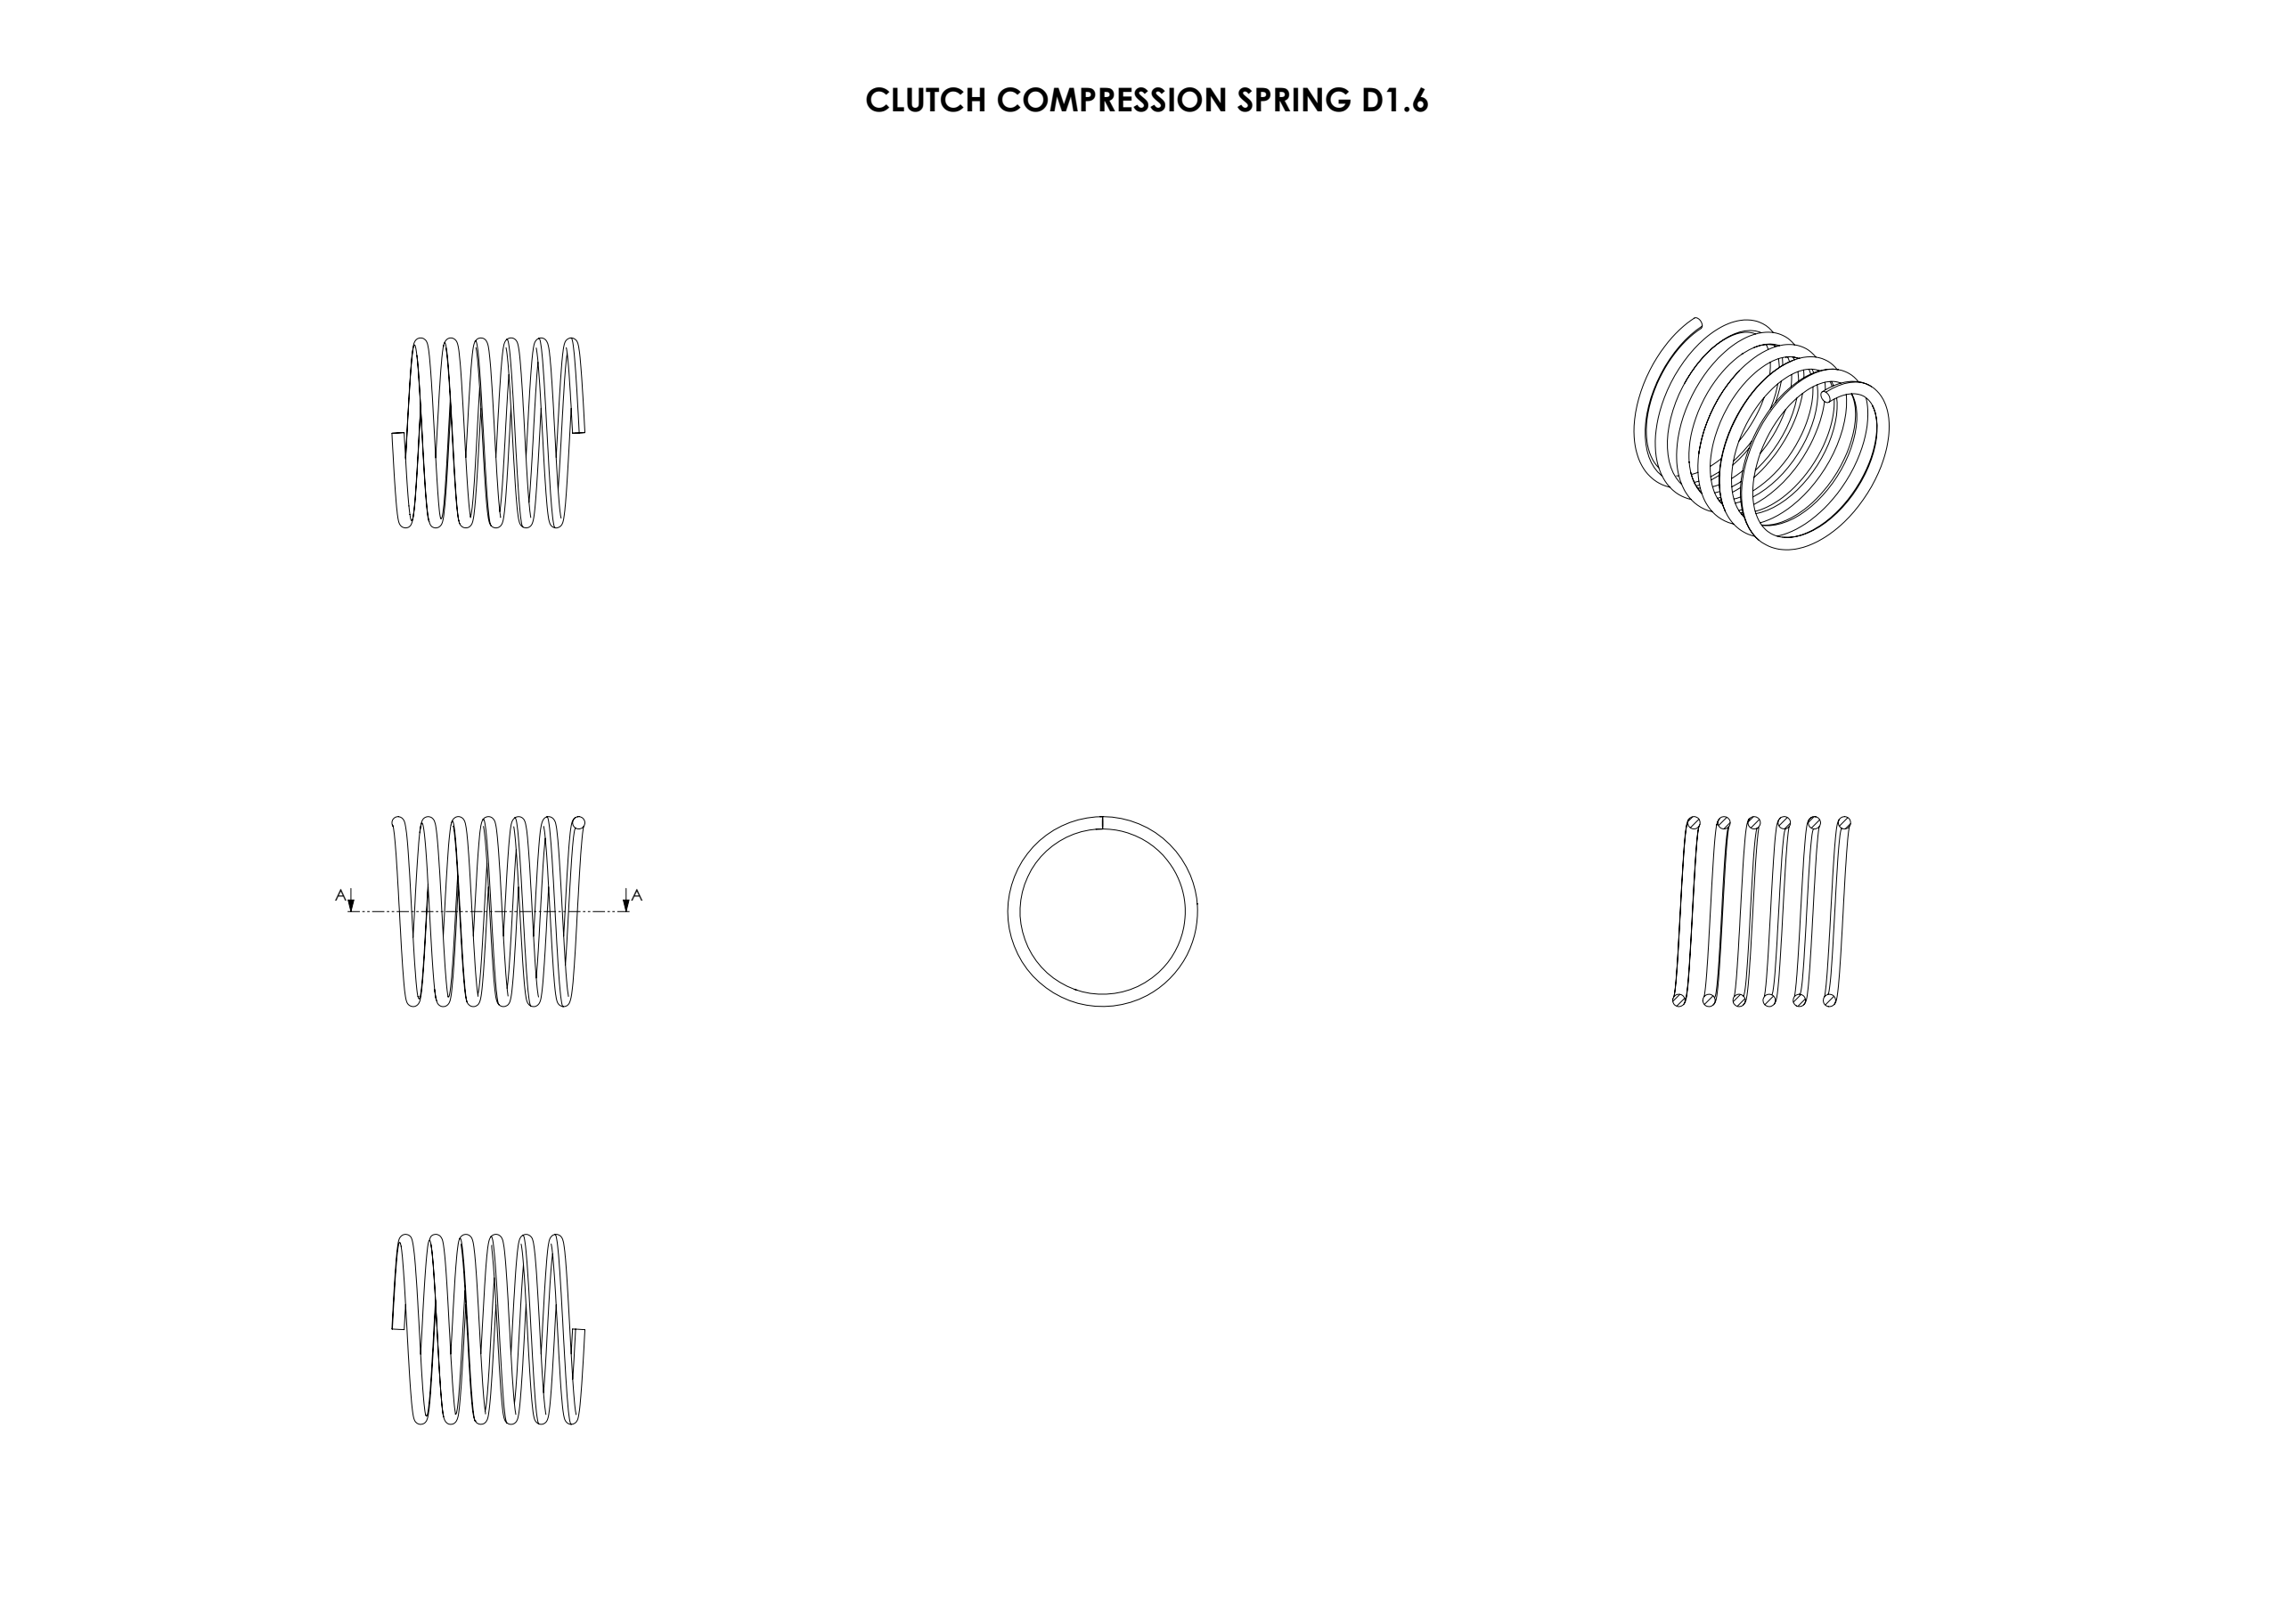
ISO-10303-21;
HEADER;
/* Generated by software containing ST-Developer
 * from STEP Tools, Inc. (www.steptools.com) 
 */

FILE_DESCRIPTION(
/* description */ (''),
/* implementation_level */ '2;1');

FILE_NAME(
/* name */ '10_Clutch_Compression_Spring_d1.6.step',
/* time_stamp */ '2026-10-11T13:00:10-07:00',
/* author */ (''),
/* organization */ (''),
/* preprocessor_version */ 'ST-DEVELOPER v20.2',
/* originating_system */ 'Autodesk Translation Framework v15.15.0.0',
/* authorisation */ '');

FILE_SCHEMA (('AUTOMOTIVE_DESIGN { 1 0 10303 214 3 1 1 }'));
ENDSEC;

DATA;
#10=MECHANICAL_DESIGN_GEOMETRIC_PRESENTATION_REPRESENTATION('',(#367),#65563);
#345=SHAPE_REPRESENTATION_RELATIONSHIP('SRR','None',#65623,#356);
#356=ADVANCED_BREP_SHAPE_REPRESENTATION('',(#378),#65561);
#367=STYLED_ITEM('',(#65788),#378);
#378=MANIFOLD_SOLID_BREP('Body1',#20017);
#843=B_SPLINE_SURFACE_WITH_KNOTS('',3,3,((#62685,#62686,#62687,#62688,#62689,
#62690,#62691,#62692,#62693,#62694,#62695,#62696,#62697,#62698,#62699,#62700,
#62701,#62702,#62703,#62704,#62705,#62706,#62707,#62708,#62709,#62710,#62711,
#62712,#62713,#62714,#62715,#62716,#62717,#62718,#62719,#62720,#62721,#62722,
#62723,#62724,#62725,#62726,#62727,#62728,#62729,#62730,#62731,#62732,#62733,
#62734,#62735,#62736,#62737,#62738,#62739,#62740,#62741,#62742,#62743,#62744,
#62745,#62746,#62747,#62748,#62749,#62750,#62751,#62752,#62753,#62754,#62755,
#62756,#62757,#62758,#62759,#62760),(#62761,#62762,#62763,#62764,#62765,
#62766,#62767,#62768,#62769,#62770,#62771,#62772,#62773,#62774,#62775,#62776,
#62777,#62778,#62779,#62780,#62781,#62782,#62783,#62784,#62785,#62786,#62787,
#62788,#62789,#62790,#62791,#62792,#62793,#62794,#62795,#62796,#62797,#62798,
#62799,#62800,#62801,#62802,#62803,#62804,#62805,#62806,#62807,#62808,#62809,
#62810,#62811,#62812,#62813,#62814,#62815,#62816,#62817,#62818,#62819,#62820,
#62821,#62822,#62823,#62824,#62825,#62826,#62827,#62828,#62829,#62830,#62831,
#62832,#62833,#62834,#62835,#62836),(#62837,#62838,#62839,#62840,#62841,
#62842,#62843,#62844,#62845,#62846,#62847,#62848,#62849,#62850,#62851,#62852,
#62853,#62854,#62855,#62856,#62857,#62858,#62859,#62860,#62861,#62862,#62863,
#62864,#62865,#62866,#62867,#62868,#62869,#62870,#62871,#62872,#62873,#62874,
#62875,#62876,#62877,#62878,#62879,#62880,#62881,#62882,#62883,#62884,#62885,
#62886,#62887,#62888,#62889,#62890,#62891,#62892,#62893,#62894,#62895,#62896,
#62897,#62898,#62899,#62900,#62901,#62902,#62903,#62904,#62905,#62906,#62907,
#62908,#62909,#62910,#62911,#62912),(#62913,#62914,#62915,#62916,#62917,
#62918,#62919,#62920,#62921,#62922,#62923,#62924,#62925,#62926,#62927,#62928,
#62929,#62930,#62931,#62932,#62933,#62934,#62935,#62936,#62937,#62938,#62939,
#62940,#62941,#62942,#62943,#62944,#62945,#62946,#62947,#62948,#62949,#62950,
#62951,#62952,#62953,#62954,#62955,#62956,#62957,#62958,#62959,#62960,#62961,
#62962,#62963,#62964,#62965,#62966,#62967,#62968,#62969,#62970,#62971,#62972,
#62973,#62974,#62975,#62976,#62977,#62978,#62979,#62980,#62981,#62982,#62983,
#62984,#62985,#62986,#62987,#62988),(#62989,#62990,#62991,#62992,#62993,
#62994,#62995,#62996,#62997,#62998,#62999,#63000,#63001,#63002,#63003,#63004,
#63005,#63006,#63007,#63008,#63009,#63010,#63011,#63012,#63013,#63014,#63015,
#63016,#63017,#63018,#63019,#63020,#63021,#63022,#63023,#63024,#63025,#63026,
#63027,#63028,#63029,#63030,#63031,#63032,#63033,#63034,#63035,#63036,#63037,
#63038,#63039,#63040,#63041,#63042,#63043,#63044,#63045,#63046,#63047,#63048,
#63049,#63050,#63051,#63052,#63053,#63054,#63055,#63056,#63057,#63058,#63059,
#63060,#63061,#63062,#63063,#63064),(#63065,#63066,#63067,#63068,#63069,
#63070,#63071,#63072,#63073,#63074,#63075,#63076,#63077,#63078,#63079,#63080,
#63081,#63082,#63083,#63084,#63085,#63086,#63087,#63088,#63089,#63090,#63091,
#63092,#63093,#63094,#63095,#63096,#63097,#63098,#63099,#63100,#63101,#63102,
#63103,#63104,#63105,#63106,#63107,#63108,#63109,#63110,#63111,#63112,#63113,
#63114,#63115,#63116,#63117,#63118,#63119,#63120,#63121,#63122,#63123,#63124,
#63125,#63126,#63127,#63128,#63129,#63130,#63131,#63132,#63133,#63134,#63135,
#63136,#63137,#63138,#63139,#63140),(#63141,#63142,#63143,#63144,#63145,
#63146,#63147,#63148,#63149,#63150,#63151,#63152,#63153,#63154,#63155,#63156,
#63157,#63158,#63159,#63160,#63161,#63162,#63163,#63164,#63165,#63166,#63167,
#63168,#63169,#63170,#63171,#63172,#63173,#63174,#63175,#63176,#63177,#63178,
#63179,#63180,#63181,#63182,#63183,#63184,#63185,#63186,#63187,#63188,#63189,
#63190,#63191,#63192,#63193,#63194,#63195,#63196,#63197,#63198,#63199,#63200,
#63201,#63202,#63203,#63204,#63205,#63206,#63207,#63208,#63209,#63210,#63211,
#63212,#63213,#63214,#63215,#63216),(#63217,#63218,#63219,#63220,#63221,
#63222,#63223,#63224,#63225,#63226,#63227,#63228,#63229,#63230,#63231,#63232,
#63233,#63234,#63235,#63236,#63237,#63238,#63239,#63240,#63241,#63242,#63243,
#63244,#63245,#63246,#63247,#63248,#63249,#63250,#63251,#63252,#63253,#63254,
#63255,#63256,#63257,#63258,#63259,#63260,#63261,#63262,#63263,#63264,#63265,
#63266,#63267,#63268,#63269,#63270,#63271,#63272,#63273,#63274,#63275,#63276,
#63277,#63278,#63279,#63280,#63281,#63282,#63283,#63284,#63285,#63286,#63287,
#63288,#63289,#63290,#63291,#63292),(#63293,#63294,#63295,#63296,#63297,
#63298,#63299,#63300,#63301,#63302,#63303,#63304,#63305,#63306,#63307,#63308,
#63309,#63310,#63311,#63312,#63313,#63314,#63315,#63316,#63317,#63318,#63319,
#63320,#63321,#63322,#63323,#63324,#63325,#63326,#63327,#63328,#63329,#63330,
#63331,#63332,#63333,#63334,#63335,#63336,#63337,#63338,#63339,#63340,#63341,
#63342,#63343,#63344,#63345,#63346,#63347,#63348,#63349,#63350,#63351,#63352,
#63353,#63354,#63355,#63356,#63357,#63358,#63359,#63360,#63361,#63362,#63363,
#63364,#63365,#63366,#63367,#63368),(#63369,#63370,#63371,#63372,#63373,
#63374,#63375,#63376,#63377,#63378,#63379,#63380,#63381,#63382,#63383,#63384,
#63385,#63386,#63387,#63388,#63389,#63390,#63391,#63392,#63393,#63394,#63395,
#63396,#63397,#63398,#63399,#63400,#63401,#63402,#63403,#63404,#63405,#63406,
#63407,#63408,#63409,#63410,#63411,#63412,#63413,#63414,#63415,#63416,#63417,
#63418,#63419,#63420,#63421,#63422,#63423,#63424,#63425,#63426,#63427,#63428,
#63429,#63430,#63431,#63432,#63433,#63434,#63435,#63436,#63437,#63438,#63439,
#63440,#63441,#63442,#63443,#63444)),.UNSPECIFIED.,.T.,.F.,.F.,(4,1,1,1,
1,1,1,4),(4,1,1,1,1,1,1,1,1,1,1,1,1,1,1,1,1,1,1,1,1,1,1,1,1,1,1,1,1,1,1,
1,1,1,1,1,1,1,1,1,1,1,1,1,1,1,1,1,1,1,1,1,1,1,1,1,1,1,1,1,1,1,1,1,1,1,1,
1,1,1,1,1,1,4),(-3.14159265358979,-2.24399475256414,-1.34639685153848,-0.448798950512828,
0.448798950512828,1.34639685153848,2.24399475256414,3.14159265358979),(0.,
0.00892857142857143,0.0178571428571429,0.0357142857142857,0.0535714285714286,
0.0714285714285714,0.0892857142857143,0.107142857142857,0.125,0.142857142857143,
0.158730158730159,0.174603174603175,0.182539682539683,0.186507936507937,
0.19047619047619,0.202380952380952,0.214285714285714,0.226190476190476,
0.238095238095238,0.25,0.261904761904762,0.273809523809524,0.279761904761905,
0.285714285714286,0.297619047619048,0.30952380952381,0.321428571428571,
0.333333333333333,0.349206349206349,0.365079365079365,0.380952380952381,
0.396825396825397,0.412698412698413,0.428571428571429,0.436507936507937,
0.452380952380952,0.464285714285714,0.476190476190476,0.488095238095238,
0.5,0.517857142857143,0.535714285714286,0.553571428571429,0.571428571428571,
0.589285714285714,0.607142857142857,0.625,0.642857142857143,0.651785714285714,
0.660714285714286,0.678571428571428,0.696428571428571,0.714285714285714,
0.726190476190476,0.738095238095238,0.75,0.761904761904762,0.773809523809524,
0.785714285714286,0.797619047619047,0.809523809523809,0.821428571428571,
0.833333333333333,0.845238095238095,0.857142857142857,0.875,0.892857142857143,
0.910714285714286,0.928571428571429,0.946428571428571,0.964285714285714,
0.982142857142857,0.991071428571429,1.),.UNSPECIFIED.);
#1038=PLANE('',#22039);
#1039=PLANE('',#22040);
#2148=FACE_OUTER_BOUND('',#3376,.T.);
#2149=FACE_OUTER_BOUND('',#3377,.T.);
#2150=FACE_OUTER_BOUND('',#3378,.T.);
#3376=EDGE_LOOP('',(#17434,#17435,#17436,#17437));
#3377=EDGE_LOOP('',(#17438));
#3378=EDGE_LOOP('',(#17439));
#4481=CIRCLE('',#22037,0.8);
#4482=CIRCLE('',#22038,0.8);
#5356=B_SPLINE_CURVE_WITH_KNOTS('',3,(#63448,#63449,#63450,#63451,#63452,
#63453,#63454,#63455,#63456,#63457,#63458,#63459,#63460,#63461,#63462,#63463,
#63464,#63465,#63466,#63467,#63468,#63469,#63470,#63471,#63472,#63473,#63474,
#63475,#63476,#63477,#63478,#63479,#63480,#63481,#63482,#63483,#63484,#63485,
#63486,#63487,#63488,#63489,#63490,#63491,#63492,#63493,#63494,#63495,#63496,
#63497,#63498,#63499,#63500,#63501,#63502,#63503,#63504,#63505,#63506,#63507,
#63508,#63509,#63510,#63511,#63512,#63513,#63514,#63515,#63516,#63517,#63518,
#63519,#63520,#63521,#63522,#63523),.UNSPECIFIED.,.F.,.F.,(4,1,1,1,1,1,
1,1,1,1,1,1,1,1,1,1,1,1,1,1,1,1,1,1,1,1,1,1,1,1,1,1,1,1,1,1,1,1,1,1,1,1,
1,1,1,1,1,1,1,1,1,1,1,1,1,1,1,1,1,1,1,1,1,1,1,1,1,1,1,1,1,1,1,4),(0.,0.00892857142857143,
0.0178571428571429,0.0357142857142857,0.0535714285714286,0.0714285714285714,
0.0892857142857143,0.107142857142857,0.125,0.142857142857143,0.158730158730159,
0.174603174603175,0.182539682539683,0.186507936507937,0.19047619047619,
0.202380952380952,0.214285714285714,0.226190476190476,0.238095238095238,
0.25,0.261904761904762,0.273809523809524,0.279761904761905,0.285714285714286,
0.297619047619048,0.30952380952381,0.321428571428571,0.333333333333333,
0.349206349206349,0.365079365079365,0.380952380952381,0.396825396825397,
0.412698412698413,0.428571428571429,0.436507936507937,0.452380952380952,
0.464285714285714,0.476190476190476,0.488095238095238,0.5,0.517857142857143,
0.535714285714286,0.553571428571429,0.571428571428571,0.589285714285714,
0.607142857142857,0.625,0.642857142857143,0.651785714285714,0.660714285714286,
0.678571428571428,0.696428571428571,0.714285714285714,0.726190476190476,
0.738095238095238,0.75,0.761904761904762,0.773809523809524,0.785714285714286,
0.797619047619047,0.809523809523809,0.821428571428571,0.833333333333333,
0.845238095238095,0.857142857142857,0.875,0.892857142857143,0.910714285714286,
0.928571428571429,0.946428571428571,0.964285714285714,0.982142857142857,
0.991071428571429,1.),.UNSPECIFIED.);
#8857=VERTEX_POINT('',#63445);
#8858=VERTEX_POINT('',#63447);
#11750=EDGE_CURVE('',#8857,#8857,#4481,.T.);
#11751=EDGE_CURVE('',#8857,#8858,#5356,.T.);
#11752=EDGE_CURVE('',#8858,#8858,#4482,.T.);
#17434=ORIENTED_EDGE('',*,*,#11750,.T.);
#17435=ORIENTED_EDGE('',*,*,#11751,.T.);
#17436=ORIENTED_EDGE('',*,*,#11752,.F.);
#17437=ORIENTED_EDGE('',*,*,#11751,.F.);
#17438=ORIENTED_EDGE('',*,*,#11752,.T.);
#17439=ORIENTED_EDGE('',*,*,#11750,.F.);
#19844=ADVANCED_FACE('',(#2148),#843,.T.);
#19845=ADVANCED_FACE('',(#2149),#1038,.T.);
#19846=ADVANCED_FACE('',(#2150),#1039,.F.);
#20017=CLOSED_SHELL('',(#19844,#19845,#19846));
#22036=AXIS2_PLACEMENT_3D('',#62684,#26929,#26930);
#22037=AXIS2_PLACEMENT_3D('',#63446,#26931,#26932);
#22038=AXIS2_PLACEMENT_3D('',#63524,#26933,#26934);
#22039=AXIS2_PLACEMENT_3D('',#63525,#26935,#26936);
#22040=AXIS2_PLACEMENT_3D('',#63526,#26937,#26938);
#26929=DIRECTION('axis',(0.,0.,1.));
#26930=DIRECTION('refdir',(1.,0.,0.));
#26931=DIRECTION('center_axis',(0.0524864875083004,-0.00359342805144231,
0.998615169073593));
#26932=DIRECTION('ref_axis',(-0.996282959525764,0.0682093869087291,0.052609353694185));
#26933=DIRECTION('center_axis',(0.052486487479681,0.00359342804742538,0.998615169075111));
#26934=DIRECTION('ref_axis',(0.504066799442469,0.863157308043356,-0.029599379574115));
#26935=DIRECTION('center_axis',(0.052486487479681,0.00359342804742538,0.998615169075111));
#26936=DIRECTION('ref_axis',(0.504066799442469,0.863157308043356,-0.029599379574115));
#26937=DIRECTION('center_axis',(0.0524864875083004,-0.00359342805144231,
0.998615169073593));
#26938=DIRECTION('ref_axis',(-0.996282959525764,0.0682093869087291,0.052609353694185));
#62684=CARTESIAN_POINT('',(0.,0.,0.));
#62685=CARTESIAN_POINT('Ctrl Pts',(-5.40297363237939,11.445432490473,-0.042087482955348));
#62686=CARTESIAN_POINT('Ctrl Pts',(-5.33369696111111,11.4406895414653,1.27598004405306));
#62687=CARTESIAN_POINT('Ctrl Pts',(-5.19521862607164,11.0085774465653,3.79612986924071));
#62688=CARTESIAN_POINT('Ctrl Pts',(-4.91840015088629,8.49992872694836,8.36573269447326));
#62689=CARTESIAN_POINT('Ctrl Pts',(-4.57320339639667,2.77438806679843,11.967805106163));
#62690=CARTESIAN_POINT('Ctrl Pts',(-4.15990469688328,-5.28321395100969,
11.056569093912));
#62691=CARTESIAN_POINT('Ctrl Pts',(-3.747686811287,-10.9955419925911,5.33820880446098));
#62692=CARTESIAN_POINT('Ctrl Pts',(-3.33647538038886,-11.8953437286105,
-2.67607624391012));
#62693=CARTESIAN_POINT('Ctrl Pts',(-2.92629230091383,-7.61357058494829,
-9.48509907357355));
#62694=CARTESIAN_POINT('Ctrl Pts',(-2.51711411539744,-0.0352081461009456,
-12.133141923791));
#62695=CARTESIAN_POINT('Ctrl Pts',(-2.12405346851776,7.23325257089384,-9.58201967934875));
#62696=CARTESIAN_POINT('Ctrl Pts',(-1.74697035839629,11.3507348234515,-3.53593739186965));
#62697=CARTESIAN_POINT('Ctrl Pts',(-1.44594495704173,11.3410956049915,2.29151330201399));
#62698=CARTESIAN_POINT('Ctrl Pts',(-1.23555813837642,9.62414272926665,5.84190263222694));
#62699=CARTESIAN_POINT('Ctrl Pts',(-1.11543119956109,8.23345778533256,7.58643680207061));
#62700=CARTESIAN_POINT('Ctrl Pts',(-0.965350761047819,6.18988758696103,
9.48427609552777));
#62701=CARTESIAN_POINT('Ctrl Pts',(-0.755455752947343,2.59800826091561,
11.2146857757666));
#62702=CARTESIAN_POINT('Ctrl Pts',(-0.486005297879084,-2.52226170629262,
11.2131697972667));
#62703=CARTESIAN_POINT('Ctrl Pts',(-0.216964169512981,-7.12771226807027,
8.99614845847778));
#62704=CARTESIAN_POINT('Ctrl Pts',(0.051673199605982,-10.3093017586739,
5.0037967419436));
#62705=CARTESIAN_POINT('Ctrl Pts',(0.319912004204202,-11.4424452984132,
0.0352862821531482));
#62706=CARTESIAN_POINT('Ctrl Pts',(0.587759827560524,-10.3093945561263,
-4.92692882386994));
#62707=CARTESIAN_POINT('Ctrl Pts',(0.810644510337,-7.66768866486485,-8.23632315062337));
#62708=CARTESIAN_POINT('Ctrl Pts',(0.9887628738834,-4.85431418623128,-10.0009017448057));
#62709=CARTESIAN_POINT('Ctrl Pts',(1.16675569936477,-1.72248496421437,-11.0992889627176));
#62710=CARTESIAN_POINT('Ctrl Pts',(1.38901397173341,2.49959534000996,-11.0999021750131));
#62711=CARTESIAN_POINT('Ctrl Pts',(1.65535913685916,7.06073570919373,-8.90264472811187));
#62712=CARTESIAN_POINT('Ctrl Pts',(1.92134523430893,10.2082911979719,-4.95142581114747));
#62713=CARTESIAN_POINT('Ctrl Pts',(2.21649491340346,11.464268710378,0.517623581655109));
#62714=CARTESIAN_POINT('Ctrl Pts',(2.54067136572795,9.61231028484355,6.51924754582076));
#62715=CARTESIAN_POINT('Ctrl Pts',(2.89372530199723,4.26040343756882,10.7809878391944));
#62716=CARTESIAN_POINT('Ctrl Pts',(3.24620579430313,-2.5499807271206,11.2895594263092));
#62717=CARTESIAN_POINT('Ctrl Pts',(3.59813519099429,-8.45086172951072,7.88046583695986));
#62718=CARTESIAN_POINT('Ctrl Pts',(3.94952923360969,-11.4105207073045,1.7432987177926));
#62719=CARTESIAN_POINT('Ctrl Pts',(4.24193167813174,-10.5600221745821,-3.85384587814088));
#62720=CARTESIAN_POINT('Ctrl Pts',(4.53402805814432,-7.47314001623606,-8.38031426693708));
#62721=CARTESIAN_POINT('Ctrl Pts',(4.79664370266186,-3.07363708606063,-10.9230350253262));
#62722=CARTESIAN_POINT('Ctrl Pts',(5.08810557752102,2.47013445948664,-10.9134823314909));
#62723=CARTESIAN_POINT('Ctrl Pts',(5.35017440554513,6.95492422204958,-8.75633618182547));
#62724=CARTESIAN_POINT('Ctrl Pts',(5.61200361956877,10.0542035018942,-4.86537952153394));
#62725=CARTESIAN_POINT('Ctrl Pts',(5.91720482332597,11.3540414258911,0.789064544875747));
#62726=CARTESIAN_POINT('Ctrl Pts',(6.26564105547289,9.10553979339257,7.23636750926088));
#62727=CARTESIAN_POINT('Ctrl Pts',(6.65717646488775,2.59867870246558,11.321535036503));
#62728=CARTESIAN_POINT('Ctrl Pts',(7.04828730943666,-5.02094595929096,10.4607994583915));
#62729=CARTESIAN_POINT('Ctrl Pts',(7.43900933211819,-10.4395500322981,5.04208746732736));
#62730=CARTESIAN_POINT('Ctrl Pts',(7.82938055234697,-11.2946782793107,-2.56617594127693));
#62731=CARTESIAN_POINT('Ctrl Pts',(8.21943575999143,-7.22551638204153,-9.04156914965989));
#62732=CARTESIAN_POINT('Ctrl Pts',(8.60921106212656,-0.0075686889805855,
-11.5674090717167));
#62733=CARTESIAN_POINT('Ctrl Pts',(8.93382080129404,5.99528673196386,-9.45936192902959));
#62734=CARTESIAN_POINT('Ctrl Pts',(9.19340748731854,9.23614030177817,-5.81293639312917));
#62735=CARTESIAN_POINT('Ctrl Pts',(9.45293101808351,11.1142702697208,-1.3107448337562));
#62736=CARTESIAN_POINT('Ctrl Pts',(9.77723136794952,10.4154952826205,5.00401083523754));
#62737=CARTESIAN_POINT('Ctrl Pts',(10.1662605952158,5.00921490063267,10.4044353775234));
#62738=CARTESIAN_POINT('Ctrl Pts',(10.5119839322498,-1.72077939907436,11.154116840079));
#62739=CARTESIAN_POINT('Ctrl Pts',(10.8144567422258,-6.89887898300864,8.65022675987097));
#62740=CARTESIAN_POINT('Ctrl Pts',(11.0737061869649,-9.97097573622103,4.80256799145211));
#62741=CARTESIAN_POINT('Ctrl Pts',(11.332954454476,-11.0656005972151,-0.0012636146746602));
#62742=CARTESIAN_POINT('Ctrl Pts',(11.592212676988,-9.96981484505854,-4.80333442118138));
#62743=CARTESIAN_POINT('Ctrl Pts',(11.8514921790329,-6.89841951530921,-8.65513848120015));
#62744=CARTESIAN_POINT('Ctrl Pts',(12.1108041978391,-2.45923784927583,-10.7938299796143));
#62745=CARTESIAN_POINT('Ctrl Pts',(12.3701601255276,2.46836208123245,-10.7925664321256));
#62746=CARTESIAN_POINT('Ctrl Pts',(12.6295710107042,6.9094980637413,-8.65413386138286));
#62747=CARTESIAN_POINT('Ctrl Pts',(12.8890481983849,9.98316171476258,-4.8004177652554));
#62748=CARTESIAN_POINT('Ctrl Pts',(13.1486032818335,11.0817124894507,0.00909499825818533));
#62749=CARTESIAN_POINT('Ctrl Pts',(13.4082458776239,9.98216422539828,4.81540788001813));
#62750=CARTESIAN_POINT('Ctrl Pts',(13.7112804745406,6.39794424339377,9.32638055254148));
#62751=CARTESIAN_POINT('Ctrl Pts',(14.0577858522366,-0.00835395432331517,
11.5770141955486));
#62752=CARTESIAN_POINT('Ctrl Pts',(14.4478987172592,-7.23337005489467,9.04881838019601));
#62753=CARTESIAN_POINT('Ctrl Pts',(14.8383177312182,-11.3068424364633,2.56726391915326));
#62754=CARTESIAN_POINT('Ctrl Pts',(15.2291319944184,-10.4497082271469,-5.04888270590908));
#62755=CARTESIAN_POINT('Ctrl Pts',(15.6202557238013,-5.02806227013448,-10.4744930049956));
#62756=CARTESIAN_POINT('Ctrl Pts',(16.0119892870161,2.60831854215743,-11.3347514386656));
#62757=CARTESIAN_POINT('Ctrl Pts',(16.338482088023,8.02442066121112,-7.9277656209221));
#62758=CARTESIAN_POINT('Ctrl Pts',(16.6004710641513,10.3977390912262,-3.60280630418266));
#62759=CARTESIAN_POINT('Ctrl Pts',(16.7309850253063,10.8049718643827,-1.22750855798432));
#62760=CARTESIAN_POINT('Ctrl Pts',(16.796746560446,10.8094741535653,0.0236795036592751));
#62761=CARTESIAN_POINT('Ctrl Pts',(-5.38662443082758,11.6842329202395,-0.042087482955348));
#62762=CARTESIAN_POINT('Ctrl Pts',(-5.31602073284708,11.6793991178476,1.30122823777898));
#62763=CARTESIAN_POINT('Ctrl Pts',(-5.17453105309391,11.2378404310333,3.87611783187972));
#62764=CARTESIAN_POINT('Ctrl Pts',(-4.89207386432173,8.67783202920574,8.53871783783621));
#62765=CARTESIAN_POINT('Ctrl Pts',(-4.53961983973176,2.83264538933516,12.2168195484002));
#62766=CARTESIAN_POINT('Ctrl Pts',(-4.11779670190641,-5.39139693844397,
11.2859525558124));
#62767=CARTESIAN_POINT('Ctrl Pts',(-3.69704974086023,-11.2215827743621,
5.44988936613388));
#62768=CARTESIAN_POINT('Ctrl Pts',(-3.27740459014898,-12.1395545614036,
-2.72889999849327));
#62769=CARTESIAN_POINT('Ctrl Pts',(-2.8588531609028,-7.77040836600443,-9.67639362221006));
#62770=CARTESIAN_POINT('Ctrl Pts',(-2.44139968754143,-0.0388721142853535,
-12.3776586948657));
#62771=CARTESIAN_POINT('Ctrl Pts',(-2.04046215341628,7.3748814694369,-9.77518585108066));
#62772=CARTESIAN_POINT('Ctrl Pts',(-1.65589905289416,11.5736066792837,-3.60919969149015));
#62773=CARTESIAN_POINT('Ctrl Pts',(-1.34897071506894,11.563561957149,2.33231726086283));
#62774=CARTESIAN_POINT('Ctrl Pts',(-1.13450959748022,9.81333086311448,5.9513827672463));
#62775=CARTESIAN_POINT('Ctrl Pts',(-1.01206942024888,8.39587803284931,7.72948090408433));
#62776=CARTESIAN_POINT('Ctrl Pts',(-0.859108571001228,6.31309527913905,
9.66370587564346));
#62777=CARTESIAN_POINT('Ctrl Pts',(-0.645184736392552,2.65240388760526,
11.4271146010615));
#62778=CARTESIAN_POINT('Ctrl Pts',(-0.370635299740237,-2.5645957521349,
11.4254307821442));
#62779=CARTESIAN_POINT('Ctrl Pts',(-0.0965765947892482,-7.25574474773981,
9.16696825093226));
#62780=CARTESIAN_POINT('Ctrl Pts',(0.177029974179721,-10.495940553954,5.10090160620736));
#62781=CARTESIAN_POINT('Ctrl Pts',(0.450155222364603,-11.6494709439128,
0.0420395084777696));
#62782=CARTESIAN_POINT('Ctrl Pts',(0.722812894385383,-10.4960064731164,
-5.00904716447792));
#62783=CARTESIAN_POINT('Ctrl Pts',(0.949649833562332,-7.80748481493112,
-8.37685596577217));
#62784=CARTESIAN_POINT('Ctrl Pts',(1.13086935173756,-4.94518515744457,-10.1720883688267));
#62785=CARTESIAN_POINT('Ctrl Pts',(1.31193547259697,-1.75933863472017,-11.2893824118723));
#62786=CARTESIAN_POINT('Ctrl Pts',(1.53800808648294,2.53496041621199,-11.2898509308499));
#62787=CARTESIAN_POINT('Ctrl Pts',(1.80882928470653,7.17245519023224,-9.0555522803647));
#62788=CARTESIAN_POINT('Ctrl Pts',(2.07920370118388,10.3716655806418,-5.03925894158933));
#62789=CARTESIAN_POINT('Ctrl Pts',(2.37912972697024,11.6476623900761,0.518107830099377));
#62790=CARTESIAN_POINT('Ctrl Pts',(2.7084215266127,9.76615815837076,6.61394631540922));
#62791=CARTESIAN_POINT('Ctrl Pts',(3.06686380982559,4.33246375617594,10.9402548757315));
#62792=CARTESIAN_POINT('Ctrl Pts',(3.42458416068682,-2.57871836910459,11.4557472388598));
#62793=CARTESIAN_POINT('Ctrl Pts',(3.78156882350692,-8.56367510055875,7.99749077041819));
#62794=CARTESIAN_POINT('Ctrl Pts',(4.13779970244094,-11.5633896761636,1.77577652817538));
#62795=CARTESIAN_POINT('Ctrl Pts',(4.43407615107156,-10.7011768584388,-3.8951157658593));
#62796=CARTESIAN_POINT('Ctrl Pts',(4.72991998621853,-7.57473185360497,-8.4794174000976));
#62797=CARTESIAN_POINT('Ctrl Pts',(4.99579563816587,-3.12059647036658,-11.0531492863553));
#62798=CARTESIAN_POINT('Ctrl Pts',(5.29071945165254,2.48877066815634,-11.0432915057983));
#62799=CARTESIAN_POINT('Ctrl Pts',(5.55579786749363,7.02472382683712,-8.86124346251412));
#62800=CARTESIAN_POINT('Ctrl Pts',(5.82051763671242,10.1578631240965,-4.92747349510609));
#62801=CARTESIAN_POINT('Ctrl Pts',(6.12893287481644,11.4710667735206,0.786351846504364));
#62802=CARTESIAN_POINT('Ctrl Pts',(6.48086970009608,9.19948880042808,7.29767185085932));
#62803=CARTESIAN_POINT('Ctrl Pts',(6.876036093994,2.63214136512159,11.4196583755266));
#62804=CARTESIAN_POINT('Ctrl Pts',(7.2704951360562,-5.05206738614446,10.5507066000566));
#62805=CARTESIAN_POINT('Ctrl Pts',(7.664269849656,-10.5119684082973,5.08929931648977));
#62806=CARTESIAN_POINT('Ctrl Pts',(8.05739638782829,-11.3721058534257,-2.5723084615911));
#62807=CARTESIAN_POINT('Ctrl Pts',(8.44991208702215,-7.27666845581022,-9.08750535291988));
#62808=CARTESIAN_POINT('Ctrl Pts',(8.84183589581078,-0.0190233677037744,
-11.6261961433184));
#62809=CARTESIAN_POINT('Ctrl Pts',(9.16800897973602,6.01193267834016,-9.50734087777631));
#62810=CARTESIAN_POINT('Ctrl Pts',(9.42865337465075,9.26567864906491,-5.84611390760456));
#62811=CARTESIAN_POINT('Ctrl Pts',(9.68913010904725,11.1505695545849,-1.32743556288045));
#62812=CARTESIAN_POINT('Ctrl Pts',(10.01444990245,10.4487042298974,5.00670632569537));
#62813=CARTESIAN_POINT('Ctrl Pts',(10.404410400302,5.0292579730303,10.418996824966));
#62814=CARTESIAN_POINT('Ctrl Pts',(10.7506877702216,-1.71103270316429,11.1687624961623));
#62815=CARTESIAN_POINT('Ctrl Pts',(11.0534087660824,-6.89297973807507,8.66266553885666));
#62816=CARTESIAN_POINT('Ctrl Pts',(11.3127577882607,-9.96570753196438,4.81359043978792));
#62817=CARTESIAN_POINT('Ctrl Pts',(11.5719265540532,-11.0597406950972,0.0113000199644781));
#62818=CARTESIAN_POINT('Ctrl Pts',(11.8309999800597,-9.96443740908525,-4.78691623055493));
#62819=CARTESIAN_POINT('Ctrl Pts',(12.089942848211,-6.89699200645375,-8.63338332691425));
#62820=CARTESIAN_POINT('Ctrl Pts',(12.3487984396484,-2.46582258118391,-10.7678176469866));
#62821=CARTESIAN_POINT('Ctrl Pts',(12.6075197618077,2.44956273217333,-10.766340494442));
#62822=CARTESIAN_POINT('Ctrl Pts',(12.8661852362955,6.87753001040116,-8.63389160824295));
#62823=CARTESIAN_POINT('Ctrl Pts',(13.1247741476138,9.94027936125449,-4.79343295279293));
#62824=CARTESIAN_POINT('Ctrl Pts',(13.3833009319311,11.0341713583544,-0.00317416406982458));
#62825=CARTESIAN_POINT('Ctrl Pts',(13.6417781017764,9.93937775359348,4.78122924367456));
#62826=CARTESIAN_POINT('Ctrl Pts',(13.9432825257392,6.3731535080168,9.26905415030222));
#62827=CARTESIAN_POINT('Ctrl Pts',(14.2878439989708,0.00300314958158428,
11.5061588243725));
#62828=CARTESIAN_POINT('Ctrl Pts',(14.6754462417248,-7.17478563786537,8.99342192147372));
#62829=CARTESIAN_POINT('Ctrl Pts',(15.0630597522916,-11.2179471506956,2.55835488475392));
#62830=CARTESIAN_POINT('Ctrl Pts',(15.4507706640767,-10.3667041184257,-4.99673895003962));
#62831=CARTESIAN_POINT('Ctrl Pts',(15.8384977092108,-4.99174936807355,-10.3743665471522));
#62832=CARTESIAN_POINT('Ctrl Pts',(16.2265565504856,2.57263136784385,-11.2253812680671));
#62833=CARTESIAN_POINT('Ctrl Pts',(16.5497447116511,7.93342720259043,-7.8526330852735));
#62834=CARTESIAN_POINT('Ctrl Pts',(16.8089720533906,10.2814647901916,-3.57330742364719));
#62835=CARTESIAN_POINT('Ctrl Pts',(16.9379965316827,10.6841596272025,-1.22522263021414));
#62836=CARTESIAN_POINT('Ctrl Pts',(17.0030907568274,10.6886162297605,0.0132690991824951));
#62837=CARTESIAN_POINT('Ctrl Pts',(-5.58213752804996,12.1756744501656,-0.0300430479348889));
#62838=CARTESIAN_POINT('Ctrl Pts',(-5.50877812904515,12.1706519818174,1.36570302154143));
#62839=CARTESIAN_POINT('Ctrl Pts',(-5.36106226989209,11.7096936310828,4.05389952128246));
#62840=CARTESIAN_POINT('Ctrl Pts',(-5.06685484898808,9.0428635992223,8.91045562475751));
#62841=CARTESIAN_POINT('Ctrl Pts',(-4.69909942041695,2.94563865221725,12.7498701343512));
#62842=CARTESIAN_POINT('Ctrl Pts',(-4.25898293676952,-5.63608587336797,
11.7779719464893));
#62843=CARTESIAN_POINT('Ctrl Pts',(-3.81963203329655,-11.7245092162211,
5.68555235440507));
#62844=CARTESIAN_POINT('Ctrl Pts',(-3.38127989331131,-12.6839981428031,
-2.85852486490255));
#62845=CARTESIAN_POINT('Ctrl Pts',(-2.94385951041784,-8.11849627124418,
-10.1194220241074));
#62846=CARTESIAN_POINT('Ctrl Pts',(-2.50743743147879,-0.0355288229951717,
-12.9441324262393));
#62847=CARTESIAN_POINT('Ctrl Pts',(-2.08814562231316,7.71791821403956,-10.2228628918827));
#62848=CARTESIAN_POINT('Ctrl Pts',(-1.68588713127857,12.1102975092266,-3.77315273387394));
#62849=CARTESIAN_POINT('Ctrl Pts',(-1.36477227087896,12.0999643764455,2.44316120718691));
#62850=CARTESIAN_POINT('Ctrl Pts',(-1.14036484630118,10.2685685552556,6.23014691826401));
#62851=CARTESIAN_POINT('Ctrl Pts',(-1.0122386454203,8.78527999884706,8.09084634428638));
#62852=CARTESIAN_POINT('Ctrl Pts',(-0.85216987072336,6.60570228047088,10.1149895329489));
#62853=CARTESIAN_POINT('Ctrl Pts',(-0.628321429176446,2.77503882988668,
11.9603687960931));
#62854=CARTESIAN_POINT('Ctrl Pts',(-0.341007099925978,-2.68468283670305,
11.9586500930173));
#62855=CARTESIAN_POINT('Ctrl Pts',(-0.0541880283575395,-7.59440137466866,
9.59501436524506));
#62856=CARTESIAN_POINT('Ctrl Pts',(0.232133536516826,-10.9853111743879,
5.33976875825063));
#62857=CARTESIAN_POINT('Ctrl Pts',(0.517951166519818,-12.1925427115221,
0.0456306551254132));
#62858=CARTESIAN_POINT('Ctrl Pts',(0.803260682123494,-10.9854331034987,
-5.24005102588547));
#62859=CARTESIAN_POINT('Ctrl Pts',(1.04059235059325,-8.17236014711802,-8.76383928564432));
#62860=CARTESIAN_POINT('Ctrl Pts',(1.2301999694469,-5.17749816539757,-10.6422030007412));
#62861=CARTESIAN_POINT('Ctrl Pts',(1.41963543254174,-1.84431402112184,-11.8111697640491));
#62862=CARTESIAN_POINT('Ctrl Pts',(1.65610507694268,2.6477367975528,-11.811608800416));
#62863=CARTESIAN_POINT('Ctrl Pts',(1.93934686505911,7.49812591212634,-9.47468373122583));
#62864=CARTESIAN_POINT('Ctrl Pts',(2.22206455148271,10.8434401317323,-5.27473146272307));
#62865=CARTESIAN_POINT('Ctrl Pts',(2.53560960785567,12.1773347135935,0.535301325191032));
#62866=CARTESIAN_POINT('Ctrl Pts',(2.87975460475582,10.2105264526929,6.90643581380321));
#62867=CARTESIAN_POINT('Ctrl Pts',(3.25424270967884,4.53310104469524,11.4261564695298));
#62868=CARTESIAN_POINT('Ctrl Pts',(3.62777977875684,-2.68423523986195,11.9641280503083));
#62869=CARTESIAN_POINT('Ctrl Pts',(4.00036632514192,-8.93103640357327,8.35396714094425));
#62870=CARTESIAN_POINT('Ctrl Pts',(4.37200507590755,-12.0601729625909,1.86268306094367));
#62871=CARTESIAN_POINT('Ctrl Pts',(4.68091022499164,-11.1607102375445,-4.05023454867948));
#62872=CARTESIAN_POINT('Ctrl Pts',(4.98922157892821,-7.90218781464488,-8.82784028522772));
#62873=CARTESIAN_POINT('Ctrl Pts',(5.26616701679252,-3.26213222142188,-11.5085441738385));
#62874=CARTESIAN_POINT('Ctrl Pts',(5.57319492830223,2.57770964828084,-11.4977849322459));
#62875=CARTESIAN_POINT('Ctrl Pts',(5.84898620445269,7.29714668223437,-9.22715804319427));
#62876=CARTESIAN_POINT('Ctrl Pts',(6.12424703583544,10.5549795888417,-5.13618793357213));
#62877=CARTESIAN_POINT('Ctrl Pts',(6.44477147423336,11.9193648706261,0.802433581377994));
#62878=CARTESIAN_POINT('Ctrl Pts',(6.810201779699,9.55929334082063,7.56370607387037));
#62879=CARTESIAN_POINT('Ctrl Pts',(7.22014147482059,2.74520255759924,11.8389419876145));
#62880=CARTESIAN_POINT('Ctrl Pts',(7.62891578995641,-5.21837344535205,10.9369214780428));
#62881=CARTESIAN_POINT('Ctrl Pts',(8.0365379096552,-10.8696746733105,5.28195384018169));
#62882=CARTESIAN_POINT('Ctrl Pts',(8.44302223705143,-11.7575201639929,-2.64075235344257));
#62883=CARTESIAN_POINT('Ctrl Pts',(8.84838123656028,-7.52639107092263,-9.36895084697553));
#62884=CARTESIAN_POINT('Ctrl Pts',(9.25263526251976,-0.0392759205799279,
-11.9860267493518));
#62885=CARTESIAN_POINT('Ctrl Pts',(9.58859730899462,6.17283522387099,-9.80208377905409));
#62886=CARTESIAN_POINT('Ctrl Pts',(9.85684366241965,9.52142304101027,-6.03375708408332));
#62887=CARTESIAN_POINT('Ctrl Pts',(10.1247368478916,11.4597337643269,-1.38603993283289));
#62888=CARTESIAN_POINT('Ctrl Pts',(10.4589411719737,10.7372829702099,5.121580228287));
#62889=CARTESIAN_POINT('Ctrl Pts',(10.8589525646346,5.17601081871361,10.672306219655));
#62890=CARTESIAN_POINT('Ctrl Pts',(11.2136246222839,-1.72855590679122,11.4388774467827));
#62891=CARTESIAN_POINT('Ctrl Pts',(11.5233392509183,-7.03015404855583,8.87404791214989));
#62892=CARTESIAN_POINT('Ctrl Pts',(11.7883721374067,-10.1702418575688,4.93991879033325));
#62893=CARTESIAN_POINT('Ctrl Pts',(12.0529994415247,-11.2866773983137,0.0361816243266041));
#62894=CARTESIAN_POINT('Ctrl Pts',(12.3172031678835,-10.1691224548695,-4.85742315527652));
#62895=CARTESIAN_POINT('Ctrl Pts',(12.5810085730965,-7.04333516732229,-8.77595778561382));
#62896=CARTESIAN_POINT('Ctrl Pts',(12.8444122722771,-2.53358181596827,-10.9476579632121));
#62897=CARTESIAN_POINT('Ctrl Pts',(13.1074454062801,2.46392456498872,-10.9454322140739));
#62898=CARTESIAN_POINT('Ctrl Pts',(13.3700914250086,6.96015352944818,-8.77946190588175));
#62899=CARTESIAN_POINT('Ctrl Pts',(13.6323722416537,10.0663826285115,-4.88343493856922));
#62900=CARTESIAN_POINT('Ctrl Pts',(13.894296945586,11.1740422712744,-0.0296971803831297));
#62901=CARTESIAN_POINT('Ctrl Pts',(14.1558727999502,10.0654107461421,4.81229139485823));
#62902=CARTESIAN_POINT('Ctrl Pts',(14.4606573163972,6.45944618588964,9.34875999480817));
#62903=CARTESIAN_POINT('Ctrl Pts',(14.8084186207746,0.0286940154300198,
11.6049438878024));
#62904=CARTESIAN_POINT('Ctrl Pts',(15.1989659292178,-7.20343837095942,9.0707366164502));
#62905=CARTESIAN_POINT('Ctrl Pts',(15.5888271044371,-11.2684315837746,2.59648807102487));
#62906=CARTESIAN_POINT('Ctrl Pts',(15.9781003660338,-10.4114044148879,-4.98937302790091));
#62907=CARTESIAN_POINT('Ctrl Pts',(16.3666890068541,-5.02240875860095,-10.3778490907909));
#62908=CARTESIAN_POINT('Ctrl Pts',(16.75491996291,2.54609586936617,-11.2269852191641));
#62909=CARTESIAN_POINT('Ctrl Pts',(17.0776472449118,7.8986520888767,-7.8571397173543));
#62910=CARTESIAN_POINT('Ctrl Pts',(17.3361860886226,10.2399861777324,-3.5889008967425));
#62911=CARTESIAN_POINT('Ctrl Pts',(17.4647378405461,10.6409669797038,-1.24921590933198));
#62912=CARTESIAN_POINT('Ctrl Pts',(17.5296467076155,10.6454108919306,-0.0142508283097832));
#62913=CARTESIAN_POINT('Ctrl Pts',(-6.34175946120379,12.4040821855152,0.0107040337528743));
#62914=CARTESIAN_POINT('Ctrl Pts',(-6.26706179117867,12.398968093954,1.43191223271551));
#62915=CARTESIAN_POINT('Ctrl Pts',(-6.11635370620616,11.9288069117454,4.17463339171532));
#62916=CARTESIAN_POINT('Ctrl Pts',(-5.81628679876286,9.2092221886427,9.12810114140272));
#62917=CARTESIAN_POINT('Ctrl Pts',(-5.44029591289839,2.97759289791273,13.0564360914058));
#62918=CARTESIAN_POINT('Ctrl Pts',(-4.98949435753561,-5.81353510375367,
12.0632665775625));
#62919=CARTESIAN_POINT('Ctrl Pts',(-4.53841730021845,-12.0667921857124,
5.81108553319272));
#62920=CARTESIAN_POINT('Ctrl Pts',(-4.08742934584185,-13.057041864785,-2.97951654626261));
#62921=CARTESIAN_POINT('Ctrl Pts',(-3.63642773955957,-8.35245308061332,
-10.4675245804829));
#62922=CARTESIAN_POINT('Ctrl Pts',(-3.18552048891545,-0.00195865738740459,
-13.3890796953648));
#62923=CARTESIAN_POINT('Ctrl Pts',(-2.751417959208,8.0264806856427,-10.5743146210541));
#62924=CARTESIAN_POINT('Ctrl Pts',(-2.33416003624442,12.5846595571708,-3.88522073955045));
#62925=CARTESIAN_POINT('Ctrl Pts',(-2.00048088021236,12.5755296487166,2.57451200864791));
#62926=CARTESIAN_POINT('Ctrl Pts',(-1.76698407230375,10.670190652471,6.51510179427282));
#62927=CARTESIAN_POINT('Ctrl Pts',(-1.63358171760574,9.12583521912976,8.45245139042781));
#62928=CARTESIAN_POINT('Ctrl Pts',(-1.46685019792153,6.85557171288117,10.560894186678));
#62929=CARTESIAN_POINT('Ctrl Pts',(-1.2335005384759,2.86250938720469,12.4851894756634));
#62930=CARTESIAN_POINT('Ctrl Pts',(-0.933608830224655,-2.83629378794764,
12.484184502557));
#62931=CARTESIAN_POINT('Ctrl Pts',(-0.633859801053286,-7.96772149200299,
10.0146740366583));
#62932=CARTESIAN_POINT('Ctrl Pts',(-0.334278396183705,-11.5163113708967,
5.56273552772346));
#62933=CARTESIAN_POINT('Ctrl Pts',(-0.0348645255961784,-12.7817158623768,
0.0168674356443003));
#62934=CARTESIAN_POINT('Ctrl Pts',(0.264362813841201,-11.5163950507525,
-5.5269006446327));
#62935=CARTESIAN_POINT('Ctrl Pts',(0.513553405915242,-8.5631641849765,-9.22718654740676));
#62936=CARTESIAN_POINT('Ctrl Pts',(0.712806926101561,-5.41596454340597,
-11.2012236785028));
#62937=CARTESIAN_POINT('Ctrl Pts',(0.911989524646343,-1.91131413349739,
-12.4304453184779));
#62938=CARTESIAN_POINT('Ctrl Pts',(1.16082303907062,2.81564799024151,-12.4314570114187));
#62939=CARTESIAN_POINT('Ctrl Pts',(1.459193817749,7.92546878244216,-9.9702951678761));
#62940=CARTESIAN_POINT('Ctrl Pts',(1.7573216234739,11.4536360269907,-5.54174799395099));
#62941=CARTESIAN_POINT('Ctrl Pts',(2.08829138644019,12.8623669859745,0.590980361928457));
#62942=CARTESIAN_POINT('Ctrl Pts',(2.45197695065466,10.785129106603,7.32433413314867));
#62943=CARTESIAN_POINT('Ctrl Pts',(2.84823026768593,4.77857709686782,12.1078614071571));
#62944=CARTESIAN_POINT('Ctrl Pts',(3.24395222388046,-2.86735584763152,12.6791154950883));
#62945=CARTESIAN_POINT('Ctrl Pts',(3.63912043631913,-9.49342202523412,8.85119319113865));
#62946=CARTESIAN_POINT('Ctrl Pts',(4.0337213999701,-12.8170179970068,1.95940039112546));
#62947=CARTESIAN_POINT('Ctrl Pts',(4.36205345736307,-11.8618890483679,-4.32554789162836));
#62948=CARTESIAN_POINT('Ctrl Pts',(4.68999551311996,-8.3960872137632,-9.40751712592762));
#62949=CARTESIAN_POINT('Ctrl Pts',(4.98478752120831,-3.45741751832818,-12.2615793993256));
#62950=CARTESIAN_POINT('Ctrl Pts',(5.31185556491466,2.76363202170254,-12.2506035050116));
#62951=CARTESIAN_POINT('Ctrl Pts',(5.60583527334105,7.79447342695731,-9.83054973508101));
#62952=CARTESIAN_POINT('Ctrl Pts',(5.89942807060424,11.2695311402808,-5.46736710999676));
#62953=CARTESIAN_POINT('Ctrl Pts',(6.24149197480825,12.7260002736351,0.870188005253589));
#62954=CARTESIAN_POINT('Ctrl Pts',(6.63174332507484,10.2065394057231,8.09093665967303));
#62955=CARTESIAN_POINT('Ctrl Pts',(7.06983734038559,2.92500698185025,12.6606037658675));
#62956=CARTESIAN_POINT('Ctrl Pts',(7.50696568218765,-5.59098643250971,11.6968630723186));
#62957=CARTESIAN_POINT('Ctrl Pts',(7.94310322458065,-11.6380802493207,5.64685644540905));
#62958=CARTESIAN_POINT('Ctrl Pts',(8.37822412215387,-12.5890445132526,-2.83387178302892));
#62959=CARTESIAN_POINT('Ctrl Pts',(8.81230632819328,-8.05854610358395,-10.0389570413963));
#62960=CARTESIAN_POINT('Ctrl Pts',(9.24532947911908,-0.038785248132775,
-12.842590638725));
#62961=CARTESIAN_POINT('Ctrl Pts',(9.60528130639712,6.61682954666117,-10.502876810536));
#62962=CARTESIAN_POINT('Ctrl Pts',(9.89269473817186,10.2046562682575,-6.46531635211994));
#62963=CARTESIAN_POINT('Ctrl Pts',(10.1797394837133,12.2815441775112,-1.48538330475788));
#62964=CARTESIAN_POINT('Ctrl Pts',(10.5378474556428,11.5073725540162,5.48755966310341));
#62965=CARTESIAN_POINT('Ctrl Pts',(10.9664455129648,5.54866596836936,11.4347559671639));
#62966=CARTESIAN_POINT('Ctrl Pts',(11.3464036646752,-1.84798660091247,12.2556102432363));
#62967=CARTESIAN_POINT('Ctrl Pts',(11.6781166939346,-7.52600746857995,9.50851847857713));
#62968=CARTESIAN_POINT('Ctrl Pts',(11.9619245164408,-10.8882955584731,5.29569253526718));
#62969=CARTESIAN_POINT('Ctrl Pts',(12.2452108460461,-12.0832976277723,0.0461979593358211));
#62970=CARTESIAN_POINT('Ctrl Pts',(12.5279739899067,-10.8870335306923,-5.19097370078296));
#62971=CARTESIAN_POINT('Ctrl Pts',(12.8102105391723,-7.54275874293532,-9.38308321473704));
#62972=CARTESIAN_POINT('Ctrl Pts',(13.0919194206535,-2.71962628545003,-11.7053766605458));
#62973=CARTESIAN_POINT('Ctrl Pts',(13.3730967409146,2.62254510442751,-11.7027590086165));
#62974=CARTESIAN_POINT('Ctrl Pts',(13.6537434878202,7.42666913824623,-9.38811573361164));
#62975=CARTESIAN_POINT('Ctrl Pts',(13.9338570502649,10.7437663434859,-5.22710379048192));
#62976=CARTESIAN_POINT('Ctrl Pts',(14.2134367039418,11.9257320683964,-0.0462399805677666));
#62977=CARTESIAN_POINT('Ctrl Pts',(14.4924819112214,10.7427611087893,5.11889347639459));
#62978=CARTESIAN_POINT('Ctrl Pts',(14.8174102629407,6.89814482154727,9.95484178310012));
#62979=CARTESIAN_POINT('Ctrl Pts',(15.1878675784235,0.0475887665098514,
12.3570599665712));
#62980=CARTESIAN_POINT('Ctrl Pts',(15.60343011016,-7.64719333189951,9.658942786652));
#62981=CARTESIAN_POINT('Ctrl Pts',(16.0177919854228,-11.9658388446688,2.77756371508464));
#62982=CARTESIAN_POINT('Ctrl Pts',(16.4309653348316,-11.0545902282553,-5.27451592744702));
#62983=CARTESIAN_POINT('Ctrl Pts',(16.8429380715054,-5.34037028988571,-10.9839370189219));
#62984=CARTESIAN_POINT('Ctrl Pts',(17.2537589451344,2.66970311374553,-11.8825373324373));
#62985=CARTESIAN_POINT('Ctrl Pts',(17.5950843011881,8.3276981377702,-8.31584017070621));
#62986=CARTESIAN_POINT('Ctrl Pts',(17.8676474164505,10.7963199255675,-3.81611675463074));
#62987=CARTESIAN_POINT('Ctrl Pts',(18.0035957502116,11.2204164513183,-1.34196072369696));
#62988=CARTESIAN_POINT('Ctrl Pts',(18.0717719751097,11.2250840595062,-0.0448304407862714));
#62989=CARTESIAN_POINT('Ctrl Pts',(-6.99577676753807,11.952974211143,0.0434554360374288));
#62990=CARTESIAN_POINT('Ctrl Pts',(-6.92354819783309,11.9480291637448,1.41768619088611));
#62991=CARTESIAN_POINT('Ctrl Pts',(-6.7784296219674,11.4953034355832,4.0586609902612));
#62992=CARTESIAN_POINT('Ctrl Pts',(-6.48867577802364,8.87010370902588,8.84204422931722));
#62993=CARTESIAN_POINT('Ctrl Pts',(-6.12530330932051,2.84823660147519,12.6398835273164));
#62994=CARTESIAN_POINT('Ctrl Pts',(-5.68857922216732,-5.6680044099001,11.6816959347463));
#62995=CARTESIAN_POINT('Ctrl Pts',(-5.25073555922688,-11.7399831228001,
5.61456522614908));
#62996=CARTESIAN_POINT('Ctrl Pts',(-4.81200855085364,-12.7064619153397,
-2.93611368688326));
#62997=CARTESIAN_POINT('Ctrl Pts',(-4.37232938788964,-8.12271966538111,
-10.2377880044934));
#62998=CARTESIAN_POINT('Ctrl Pts',(-3.93176827936533,0.0348328210943832,
-13.0952412158728));
#62999=CARTESIAN_POINT('Ctrl Pts',(-3.50668474008689,7.89732345693862,-10.3419323625203));
#63000=CARTESIAN_POINT('Ctrl Pts',(-3.09722403722738,12.3722191925458,-3.7793768466969));
#63001=CARTESIAN_POINT('Ctrl Pts',(-2.76912452694493,12.3650890133529,2.57226891368155));
#63002=CARTESIAN_POINT('Ctrl Pts',(-2.53919306504922,10.4891472653307,6.45285596073122));
#63003=CARTESIAN_POINT('Ctrl Pts',(-2.40772900615144,8.96727281566909,8.36205471574902));
#63004=CARTESIAN_POINT('Ctrl Pts',(-2.2433365747859,6.72892811627392,10.4409303885383));
#63005=CARTESIAN_POINT('Ctrl Pts',(-2.01300451361892,2.78796532718832,12.340912648531));
#63006=CARTESIAN_POINT('Ctrl Pts',(-1.71654890422905,-2.84542392262709,
12.3409008152921));
#63007=CARTESIAN_POINT('Ctrl Pts',(-1.41978813824793,-7.92600416136757,
9.89691654580502));
#63008=CARTESIAN_POINT('Ctrl Pts',(-1.12271904140829,-11.4455308662374,
5.48309264597084));
#63009=CARTESIAN_POINT('Ctrl Pts',(-0.825363517227147,-12.7031226545021,
-0.0243048795543868));
#63010=CARTESIAN_POINT('Ctrl Pts',(-0.527731514558294,-11.4455893823448,
-5.53859048082785));
#63011=CARTESIAN_POINT('Ctrl Pts',(-0.279478005503598,-8.50418660255496,
-9.22536834241496));
#63012=CARTESIAN_POINT('Ctrl Pts',(-0.0807549704906864,-5.36547510445352,
-11.1942782947732));
#63013=CARTESIAN_POINT('Ctrl Pts',(0.118051755945107,-1.8675651818906,-12.4213082475664));
#63014=CARTESIAN_POINT('Ctrl Pts',(0.366722102791505,2.85612569879392,-12.4231343878714));
#63015=CARTESIAN_POINT('Ctrl Pts',(0.665352877801153,7.97071605146552,-9.96078604555384));
#63016=CARTESIAN_POINT('Ctrl Pts',(0.964206395126258,11.5081607160169,-5.52218356455426));
#63017=CARTESIAN_POINT('Ctrl Pts',(1.29649977104871,12.9235881289301,0.634564968811868));
#63018=CARTESIAN_POINT('Ctrl Pts',(1.66230004176491,10.8364263379226,7.40750400995353));
#63019=CARTESIAN_POINT('Ctrl Pts',(2.06167174932048,4.78420119573235,12.230536232645));
#63020=CARTESIAN_POINT('Ctrl Pts',(2.4613476543818,-2.93770395852455,12.8098037984882));
#63021=CARTESIAN_POINT('Ctrl Pts',(2.86128398965418,-9.64464038610263,8.93787022257689));
#63022=CARTESIAN_POINT('Ctrl Pts',(3.26144748282469,-13.0171740913694,1.95011291304442));
#63023=CARTESIAN_POINT('Ctrl Pts',(3.59508775314631,-12.0484781972671,-4.43660651624035));
#63024=CARTESIAN_POINT('Ctrl Pts',(3.92883523912539,-8.52186871803321,-9.60879315096172));
#63025=CARTESIAN_POINT('Ctrl Pts',(4.22929904502273,-3.48912056106834,-12.5190732399397));
#63026=CARTESIAN_POINT('Ctrl Pts',(4.56323741679503,2.86256934376227,-12.5090759805677));
#63027=CARTESIAN_POINT('Ctrl Pts',(4.86384381459426,8.00709959101652,-10.0353408515575));
#63028=CARTESIAN_POINT('Ctrl Pts',(5.16449854937864,11.5664022511167,-5.56793348942886));
#63029=CARTESIAN_POINT('Ctrl Pts',(5.51529547561481,13.0611497278196,0.930947571039876));
#63030=CARTESIAN_POINT('Ctrl Pts',(5.91625229346491,10.4753825672146,8.35038622910933));
#63031=CARTESIAN_POINT('Ctrl Pts',(6.36731990925114,2.98011034179285,13.0580379108325));
#63032=CARTESIAN_POINT('Ctrl Pts',(6.81834949067038,-5.80685122812227,12.0668130502114));
#63033=CARTESIAN_POINT('Ctrl Pts',(7.26929377330161,-12.0612898991556,5.81375475793947));
#63034=CARTESIAN_POINT('Ctrl Pts',(7.72010735706853,-13.0495675260762,-2.97232521957111));
#63035=CARTESIAN_POINT('Ctrl Pts',(8.17075036739142,-8.34884614818407,-10.4536677858431));
#63036=CARTESIAN_POINT('Ctrl Pts',(8.62117589579843,-0.00791391267151051,
-13.3727411912355));
#63037=CARTESIAN_POINT('Ctrl Pts',(8.99632517267344,6.92934274946376,-10.936465798048));
#63038=CARTESIAN_POINT('Ctrl Pts',(9.29628043819794,10.6740986744864,-6.72296849065872));
#63039=CARTESIAN_POINT('Ctrl Pts',(9.59612919106517,12.8440088694065,-1.52123511579387));
#63040=CARTESIAN_POINT('Ctrl Pts',(9.97073190268916,12.0363481832331,5.77286443669366));
#63041=CARTESIAN_POINT('Ctrl Pts',(10.4198783301282,5.79407206251631,12.0070815806333));
#63042=CARTESIAN_POINT('Ctrl Pts',(10.8187411384565,-1.97027233311315,12.8708724365812));
#63043=CARTESIAN_POINT('Ctrl Pts',(11.1674340824346,-7.93932119118973,9.98396585791531));
#63044=CARTESIAN_POINT('Ctrl Pts',(11.4661029846676,-11.4780906888311,5.55105116774377));
#63045=CARTESIAN_POINT('Ctrl Pts',(11.7645290272056,-12.7376376654062,0.0211894625936921));
#63046=CARTESIAN_POINT('Ctrl Pts',(12.0627229130648,-11.4767297176299,-5.50183090606377));
#63047=CARTESIAN_POINT('Ctrl Pts',(12.3606592012589,-7.94698392227365,-9.92748510239363));
#63048=CARTESIAN_POINT('Ctrl Pts',(12.6583360267427,-2.8508280855602,-12.3819217266038));
#63049=CARTESIAN_POINT('Ctrl Pts',(12.9557247677888,2.79931904143353,-12.379773222104));
#63050=CARTESIAN_POINT('Ctrl Pts',(13.2528343635669,7.88544101719467,-9.92990805014466));
#63051=CARTESIAN_POINT('Ctrl Pts',(13.549644270199,11.4006534463597,-5.52129050887731));
#63052=CARTESIAN_POINT('Ctrl Pts',(13.8461441282306,12.6546960389499,-0.0270590683343575));
#63053=CARTESIAN_POINT('Ctrl Pts',(14.142325486993,11.3995925558707,5.45532204259041));
#63054=CARTESIAN_POINT('Ctrl Pts',(14.4874806409761,7.31619812550857,10.5926204476333));
#63055=CARTESIAN_POINT('Ctrl Pts',(14.8813899261482,0.0326555994906588,
13.1482752638617));
#63056=CARTESIAN_POINT('Ctrl Pts',(15.3237262854681,-8.15850127667032,10.2777019802623));
#63057=CARTESIAN_POINT('Ctrl Pts',(15.7652478499986,-12.7611663516314,2.94651360079951));
#63058=CARTESIAN_POINT('Ctrl Pts',(16.2058751260915,-11.7908725563387,-5.6416476886062));
#63059=CARTESIAN_POINT('Ctrl Pts',(16.6456846506483,-5.69172965589703,-11.7358279093178));
#63060=CARTESIAN_POINT('Ctrl Pts',(17.084418208847,2.86369100930359,-12.6988551400737));
#63061=CARTESIAN_POINT('Ctrl Pts',(17.4495345059912,8.91441846626095,-8.88278736054426));
#63062=CARTESIAN_POINT('Ctrl Pts',(17.7406676458964,11.5522099350677,-4.07665772399991));
#63063=CARTESIAN_POINT('Ctrl Pts',(17.8865302419488,12.0072646015869,-1.42218653131724));
#63064=CARTESIAN_POINT('Ctrl Pts',(17.9590854976129,12.0122320151672,-0.0417402034811674));
#63065=CARTESIAN_POINT('Ctrl Pts',(-7.04836243219494,11.1602873706909,0.0433668871147811));
#63066=CARTESIAN_POINT('Ctrl Pts',(-6.98054923009834,11.1556446164462,1.33359024729692));
#63067=CARTESIAN_POINT('Ctrl Pts',(-6.84542083169465,10.734108144334,3.79280974414481));
#63068=CARTESIAN_POINT('Ctrl Pts',(-6.57440587453761,8.27955737620748,8.26700195680993));
#63069=CARTESIAN_POINT('Ctrl Pts',(-6.23509541011525,2.6547559310062,11.8124549780299));
#63070=CARTESIAN_POINT('Ctrl Pts',(-5.82667850202676,-5.30836037069009,
10.9193453075009));
#63071=CARTESIAN_POINT('Ctrl Pts',(-5.41714811934068,-10.9886329727755,
5.24339954566476));
#63072=CARTESIAN_POINT('Ctrl Pts',(-5.00642724205123,-11.8945997983615,
-2.76045718501004));
#63073=CARTESIAN_POINT('Ctrl Pts',(-4.5945364954459,-7.60126338096456,-9.60168441536687));
#63074=CARTESIAN_POINT('Ctrl Pts',(-4.18145490797301,0.0469804373507585,
-12.2819941081016));
#63075=CARTESIAN_POINT('Ctrl Pts',(-3.78252541805809,7.42629200691454,-9.69929592859116));
#63076=CARTESIAN_POINT('Ctrl Pts',(-3.39789099794522,11.6308417690081,-3.53519632822153));
#63077=CARTESIAN_POINT('Ctrl Pts',(-3.08939324254413,11.6250000259672,2.43710008693653));
#63078=CARTESIAN_POINT('Ctrl Pts',(-2.87302899057922,9.85989537087712,6.08882885264012));
#63079=CARTESIAN_POINT('Ctrl Pts',(-2.74927343717844,8.42726546917283,7.88610073971078));
#63080=CARTESIAN_POINT('Ctrl Pts',(-2.5944799794377,6.3196412110271,9.84362143917224));
#63081=CARTESIAN_POINT('Ctrl Pts',(-2.37749287855617,2.60710207818047,11.6339173336133));
#63082=CARTESIAN_POINT('Ctrl Pts',(-2.09797454340211,-2.70450448853709,
11.6344255830779));
#63083=CARTESIAN_POINT('Ctrl Pts',(-1.81792170554395,-7.49931778606355,
9.32850799058278));
#63084=CARTESIAN_POINT('Ctrl Pts',(-1.53733736459604,-10.8240376978191,
5.15986381030307));
#63085=CARTESIAN_POINT('Ctrl Pts',(-1.2562206918343,-12.0135545707024,-0.0467397984840756));
#63086=CARTESIAN_POINT('Ctrl Pts',(-0.974573862808477,-10.8241045261154,
-5.26507248654322));
#63087=CARTESIAN_POINT('Ctrl Pts',(-0.739428880773772,-8.03834277864345,
-8.7575825674062));
#63088=CARTESIAN_POINT('Ctrl Pts',(-0.551047584316217,-5.0629822009722,
-10.6241459120783));
#63089=CARTESIAN_POINT('Ctrl Pts',(-0.36249111019426,-1.74543644090898,
-11.7880199128214));
#63090=CARTESIAN_POINT('Ctrl Pts',(-0.126471246010493,2.73805411019759,
-11.7902852668568));
#63091=CARTESIAN_POINT('Ctrl Pts',(0.15727512594571,7.59811342657792,-9.45125426124965));
#63092=CARTESIAN_POINT('Ctrl Pts',(0.441539765519954,10.9634581264468,-5.22961150140885));
#63093=CARTESIAN_POINT('Ctrl Pts',(0.757961052591613,12.3120920790573,0.632947183835009));
#63094=CARTESIAN_POINT('Ctrl Pts',(1.106753006709,10.3234214073197,7.09159088554642));
#63095=CARTESIAN_POINT('Ctrl Pts',(1.48815637392869,4.54447620677922,11.6990671932346));
#63096=CARTESIAN_POINT('Ctrl Pts',(1.87044320169088,-2.84159511207509,12.2549877464399));
#63097=CARTESIAN_POINT('Ctrl Pts',(2.25360605983208,-9.26834602877216,8.54689771165241));
#63098=CARTESIAN_POINT('Ctrl Pts',(2.63764130942004,-12.506791768106,1.84154262526316));
#63099=CARTESIAN_POINT('Ctrl Pts',(2.95837917353033,-11.5770968607523,-4.29863956570323));
#63100=CARTESIAN_POINT('Ctrl Pts',(3.27964083689423,-8.18273565833188,-9.27768576125995));
#63101=CARTESIAN_POINT('Ctrl Pts',(3.56924420355609,-3.33250795673198,-12.0840904780873));
#63102=CARTESIAN_POINT('Ctrl Pts',(3.89162245652149,2.79949587180547,-12.075394977273));
#63103=CARTESIAN_POINT('Ctrl Pts',(4.18221107033807,7.77306303674672,-9.68479374718664));
#63104=CARTESIAN_POINT('Ctrl Pts',(4.47324550024543,11.2192354884859,-5.36069128118948));
#63105=CARTESIAN_POINT('Ctrl Pts',(4.81329994937238,12.6692418509689,0.938993978829623));
#63106=CARTESIAN_POINT('Ctrl Pts',(5.20264288309048,10.1607760172556,8.1446283728886));
#63107=CARTESIAN_POINT('Ctrl Pts',(5.64159910107618,2.86826488077924,12.7287442963195));
#63108=CARTESIAN_POINT('Ctrl Pts',(6.08146878975716,-5.70197123211863,11.7651487592271));
#63109=CARTESIAN_POINT('Ctrl Pts',(6.52222468717438,-11.8175960823832,5.65548456063045));
#63110=CARTESIAN_POINT('Ctrl Pts',(6.9638341956865,-12.7890005253937,-2.9511346052465));
#63111=CARTESIAN_POINT('Ctrl Pts',(7.406265245255,-8.17660276171336,-10.2982067424904));
#63112=CARTESIAN_POINT('Ctrl Pts',(7.84949033536914,0.0301268930120722,
-13.1738913494456));
#63113=CARTESIAN_POINT('Ctrl Pts',(8.21946795867107,6.8730544511525,-10.773707415888));
#63114=CARTESIAN_POINT('Ctrl Pts',(8.51582239217239,10.5734673348988,-6.61096540438714));
#63115=CARTESIAN_POINT('Ctrl Pts',(8.81241356784579,12.7202653194831,-1.46599044540228));
#63116=CARTESIAN_POINT('Ctrl Pts',(9.18357435136159,11.92282528886,5.76150100397621));
#63117=CARTESIAN_POINT('Ctrl Pts',(9.62961377853879,5.72592863888784,11.9553621584614));
#63118=CARTESIAN_POINT('Ctrl Pts',(10.0266360172958,-2.00273443034567,12.8182691334911));
#63119=CARTESIAN_POINT('Ctrl Pts',(10.3744160574443,-7.95691351092337,9.93987207302513));
#63120=CARTESIAN_POINT('Ctrl Pts',(10.6727487589153,-11.4926568425675,5.51240413664081));
#63121=CARTESIAN_POINT('Ctrl Pts',(10.9713288571319,-12.7538129729755,-0.0201879333039461));
#63122=CARTESIAN_POINT('Ctrl Pts',(11.2701178023546,-11.4913614123974,-5.55469829188671));
#63123=CARTESIAN_POINT('Ctrl Pts',(11.5691210946344,-7.94962366264769,-9.99691887323886));
#63124=CARTESIAN_POINT('Ctrl Pts',(11.8683146332215,-2.82771967206129,-12.4649155906732));
#63125=CARTESIAN_POINT('Ctrl Pts',(12.1677087571372,2.86064740523475,-12.4636884231645));
#63126=CARTESIAN_POINT('Ctrl Pts',(12.4672656194031,7.98928703920157,-9.99446720376893));
#63127=CARTESIAN_POINT('Ctrl Pts',(12.7669854736347,11.539839877033,-5.54307362452573));
#63128=CARTESIAN_POINT('Ctrl Pts',(13.0668545363388,12.8091293590171,0.0135521506018108));
#63129=CARTESIAN_POINT('Ctrl Pts',(13.3668611248283,11.5386673942862,5.56715714768572));
#63130=CARTESIAN_POINT('Ctrl Pts',(13.7170156480823,7.39700058178498,10.7796506199623));
#63131=CARTESIAN_POINT('Ctrl Pts',(14.1173696451114,-0.00500635456861792,
13.3799462588683));
#63132=CARTESIAN_POINT('Ctrl Pts',(14.5679743207715,-8.35073144806058,10.4588250356471));
#63133=CARTESIAN_POINT('Ctrl Pts',(15.0187604015418,-13.0529116373161,2.97536203022895));
#63134=CARTESIAN_POINT('Ctrl Pts',(15.4696255793761,-12.0633772300983,-5.81330552308052));
#63135=CARTESIAN_POINT('Ctrl Pts',(15.9206676140184,-5.81066798050118,-12.0651133483454));
#63136=CARTESIAN_POINT('Ctrl Pts',(16.3715292508672,2.98158699450849,-13.0587842802026));
#63137=CARTESIAN_POINT('Ctrl Pts',(16.74763550258,9.21538084923311,-9.12936080720287));
#63138=CARTESIAN_POINT('Ctrl Pts',(17.0478498402495,11.9363656394525,-4.17344447879534));
#63139=CARTESIAN_POINT('Ctrl Pts',(17.1986488358564,12.4067864910178,-1.42910559164386));
#63140=CARTESIAN_POINT('Ctrl Pts',(17.2733863906656,12.4119033132428,-0.00713853848606688));
#63141=CARTESIAN_POINT('Ctrl Pts',(-6.46451084474973,10.6219998496075,0.0107430921454236));
#63142=CARTESIAN_POINT('Ctrl Pts',(-6.39973786109817,10.6175652404827,1.24312283579603));
#63143=CARTESIAN_POINT('Ctrl Pts',(-6.27148773155715,10.2175233413502,3.57725363696463));
#63144=CARTESIAN_POINT('Ctrl Pts',(-6.01354281718277,7.88152801963195,7.83570282159969));
#63145=CARTESIAN_POINT('Ctrl Pts',(-5.6916402210612,2.54243119535446,11.1966519138041));
#63146=CARTESIAN_POINT('Ctrl Pts',(-5.30446195420775,-5.00545208161645,
10.3497136548024));
#63147=CARTESIAN_POINT('Ctrl Pts',(-4.91701686110735,-10.378305483713,4.97667753500867));
#63148=CARTESIAN_POINT('Ctrl Pts',(-4.52896396181057,-11.2325118891829,
-2.5850252195442));
#63149=CARTESIAN_POINT('Ctrl Pts',(-4.14040222720135,-7.18047154399281,
-9.03829370587454));
#63150=CARTESIAN_POINT('Ctrl Pts',(-3.75123335740469,0.0256095269495808,
-11.5617311438726));
#63151=CARTESIAN_POINT('Ctrl Pts',(-3.37588434017118,6.96841646516042,-9.13023292284201));
#63152=CARTESIAN_POINT('Ctrl Pts',(-3.01438757125082,10.9191588748908,-3.336215850523));
#63153=CARTESIAN_POINT('Ctrl Pts',(-2.72473343890907,10.9128857663664,2.27133764692916));
#63154=CARTESIAN_POINT('Ctrl Pts',(-2.52171757764907,9.25656237679485,5.69770180441265));
#63155=CARTESIAN_POINT('Ctrl Pts',(-2.40563491295491,7.9127356846986,7.38354185859245));
#63156=CARTESIAN_POINT('Ctrl Pts',(-2.2604702649357,5.93618622336592,9.21928819606915));
#63157=CARTESIAN_POINT('Ctrl Pts',(-2.05707464492104,2.456009344374,10.8972276117971));
#63158=CARTESIAN_POINT('Ctrl Pts',(-1.79521358272284,-2.5200959412735,10.8973620123061));
#63159=CARTESIAN_POINT('Ctrl Pts',(-1.53299186318285,-7.00951239375684,
8.73797920866642));
#63160=CARTESIAN_POINT('Ctrl Pts',(-1.27041014228868,-10.1206970399566,
4.83657004935519));
#63161=CARTESIAN_POINT('Ctrl Pts',(-1.00745089130815,-11.2331352219311,
-0.0338319676480412));
#63162=CARTESIAN_POINT('Ctrl Pts',(-0.744106125260249,-10.1207240761438,
-4.91302292482435));
#63163=CARTESIAN_POINT('Ctrl Pts',(-0.524326291037735,-7.51683671547534,
-8.1772128104801));
#63164=CARTESIAN_POINT('Ctrl Pts',(-0.348297896955578,-4.73656341431799,
-9.9213468149702));
#63165=CARTESIAN_POINT('Ctrl Pts',(-0.172134410376588,-1.63704484364765,
-11.0086906838672));
#63166=CARTESIAN_POINT('Ctrl Pts',(0.0483231360515193,2.55082881753386,
-11.0106551516741));
#63167=CARTESIAN_POINT('Ctrl Pts',(0.313293760511986,7.08920053100004,-8.82626877853864));
#63168=CARTESIAN_POINT('Ctrl Pts',(0.578689934519355,10.2310632724682,-4.88476898925453));
#63169=CARTESIAN_POINT('Ctrl Pts',(0.874057039176359,11.4898322642623,0.587734432288766));
#63170=CARTESIAN_POINT('Ctrl Pts',(1.19959272293443,9.63362448009566,6.61561806556494));
#63171=CARTESIAN_POINT('Ctrl Pts',(1.55552459185528,4.24058903205902,10.9153192716146));
#63172=CARTESIAN_POINT('Ctrl Pts',(1.91227491147004,-2.6520217183213,11.4340475330235));
#63173=CARTESIAN_POINT('Ctrl Pts',(2.26986112049208,-8.64968231974067,7.97358806105671));
#63174=CARTESIAN_POINT('Ctrl Pts',(2.62829340991396,-11.6723112697667,1.71535743622179));
#63175=CARTESIAN_POINT('Ctrl Pts',(2.92770617853484,-10.804591364036,-4.01651813335133));
#63176=CARTESIAN_POINT('Ctrl Pts',(3.22766556999648,-7.63540278102332,-8.66538451201058));
#63177=CARTESIAN_POINT('Ctrl Pts',(3.4981240761088,-3.10596760239311,-11.2864014018338));
#63178=CARTESIAN_POINT('Ctrl Pts',(3.79928270555332,2.62235242391335,-11.2784987560585));
#63179=CARTESIAN_POINT('Ctrl Pts',(4.07083363394759,7.27005370883939,-9.04470812959211));
#63180=CARTESIAN_POINT('Ctrl Pts',(4.34289415231203,10.4916521068476,-5.0027262212335));
#63181=CARTESIAN_POINT('Ctrl Pts',(4.66089571348296,11.8478670218135,0.888232375739401));
#63182=CARTESIAN_POINT('Ctrl Pts',(5.02519340925734,9.50159493778667,7.6303760718029));
#63183=CARTESIAN_POINT('Ctrl Pts',(5.43620055799739,2.67414369723583,11.9233586539389));
#63184=CARTESIAN_POINT('Ctrl Pts',(5.8483918643095,-5.35671023029638,11.0215334211548));
#63185=CARTESIAN_POINT('Ctrl Pts',(6.26177439049753,-11.0932021843605,5.292365326979));
#63186=CARTESIAN_POINT('Ctrl Pts',(6.67635400543509,-12.0064745014867,-2.78707182970431));
#63187=CARTESIAN_POINT('Ctrl Pts',(7.09213698834625,-7.67323447007579,-9.69208842969653));
#63188=CARTESIAN_POINT('Ctrl Pts',(7.50912165860666,0.0468454391472405,
-12.3989463730217));
#63189=CARTESIAN_POINT('Ctrl Pts',(7.85762186683386,6.49272731621592,-10.1394282360524));
#63190=CARTESIAN_POINT('Ctrl Pts',(8.1370130781375,9.98148681853618,-6.21518078295535));
#63191=CARTESIAN_POINT('Ctrl Pts',(8.41680490762239,12.006925113785,-1.36188908633659));
#63192=CARTESIAN_POINT('Ctrl Pts',(8.76730393267241,11.2553288749941,5.46305292595075));
#63193=CARTESIAN_POINT('Ctrl Pts',(9.18910851961994,5.39694230000765,11.3216601465911));
#63194=CARTESIAN_POINT('Ctrl Pts',(9.56511020248836,-1.92199990529629,12.1404778976687));
#63195=CARTESIAN_POINT('Ctrl Pts',(9.8948686207416,-7.56786642714936,9.41200252003379));
#63196=CARTESIAN_POINT('Ctrl Pts',(10.1780547485049,-10.9243129504653,5.20988772093761));
#63197=CARTESIAN_POINT('Ctrl Pts',(10.4617475384838,-12.1232577320106,-0.0466174706278744));
#63198=CARTESIAN_POINT('Ctrl Pts',(10.7459743347294,-10.9229595673016,-5.3112508257592));
#63199=CARTESIAN_POINT('Ctrl Pts',(11.0307120599722,-7.55087576180269,-9.54183041614082));
#63200=CARTESIAN_POINT('Ctrl Pts',(11.3159714208886,-2.66808064202225,-11.8953207101883));
#63201=CARTESIAN_POINT('Ctrl Pts',(11.6017219729367,2.76095286619628,-11.8949196289229));
#63202=CARTESIAN_POINT('Ctrl Pts',(11.8879901126779,7.66215797385631,-9.53596929854585));
#63203=CARTESIAN_POINT('Ctrl Pts',(12.1747562619772,11.0596787348937,-5.27762781084655));
#63204=CARTESIAN_POINT('Ctrl Pts',(12.4620164112936,12.276330565939,0.0449487542660262));
#63205=CARTESIAN_POINT('Ctrl Pts',(12.7497675937242,11.0585470320048,5.37163302664251));
#63206=CARTESIAN_POINT('Ctrl Pts',(13.0860359161205,7.08211853912157,10.3777700655797));
#63207=CARTESIAN_POINT('Ctrl Pts',(13.4711607269014,-0.0370068386633191,
12.8813060800447));
#63208=CARTESIAN_POINT('Ctrl Pts',(13.9054671788381,-8.08136907240343,10.0687773727722));
#63209=CARTESIAN_POINT('Ctrl Pts',(14.3408246393693,-12.624968966042,2.84325776332699));
#63210=CARTESIAN_POINT('Ctrl Pts',(14.7771670529737,-11.6702358127997,-5.66182189773967));
#63211=CARTESIAN_POINT('Ctrl Pts',(15.2145608917499,-5.60909929244629,-11.7270189034878));
#63212=CARTESIAN_POINT('Ctrl Pts',(15.6527884242738,2.93550487495931,-12.6948971579645));
#63213=CARTESIAN_POINT('Ctrl Pts',(16.0190063123979,9.00736970826819,-8.87180598157205));
#63214=CARTESIAN_POINT('Ctrl Pts',(16.312038702112,11.6635526352396,-4.03468871097921));
#63215=CARTESIAN_POINT('Ctrl Pts',(16.4591456512362,12.1226664499012,-1.35766244804026));
#63216=CARTESIAN_POINT('Ctrl Pts',(16.5322293926541,12.1276700456614,0.032838922831008));
#63217=CARTESIAN_POINT('Ctrl Pts',(-5.67986690813377,10.7476981461842,-0.0300449087323375));
#63218=CARTESIAN_POINT('Ctrl Pts',(-5.61446261326135,10.7432203150502,1.2143462495032));
#63219=CARTESIAN_POINT('Ctrl Pts',(-5.48474172974139,10.338418680291,3.57512573258163));
#63220=CARTESIAN_POINT('Ctrl Pts',(-5.22429202276908,7.97900472045824,7.87465592993745));
#63221=CARTESIAN_POINT('Ctrl Pts',(-4.89987273796351,2.59696395563541,11.2594571007491));
#63222=CARTESIAN_POINT('Ctrl Pts',(-4.51074074352916,-4.98843741605642,
10.4047506337951));
#63223=CARTESIAN_POINT('Ctrl Pts',(-4.12237963223429,-10.3713388494899,
5.01690086047654));
#63224=CARTESIAN_POINT('Ctrl Pts',(-3.73446117498051,-11.2218192436182,
-2.54233631811985));
#63225=CARTESIAN_POINT('Ctrl Pts',(-3.34707792581103,-7.17929284493749,
-8.97399278959156));
#63226=CARTESIAN_POINT('Ctrl Pts',(-2.96013196535152,-0.0134791104480878,
-11.4796641361566));
#63227=CARTESIAN_POINT('Ctrl Pts',(-2.58792476469585,6.86992918584355,-9.06556804792655));
#63228=CARTESIAN_POINT('Ctrl Pts',(-2.23035369122419,10.7755084984827,-3.33320230703603));
#63229=CARTESIAN_POINT('Ctrl Pts',(-1.94452142571969,10.7674793826984,2.20014896093121));
#63230=CARTESIAN_POINT('Ctrl Pts',(-1.74454263547472,9.13565802983238,5.57501603792962));
#63231=CARTESIAN_POINT('Ctrl Pts',(-1.63029710540912,7.81308261009993,7.23414756185225));
#63232=CARTESIAN_POINT('Ctrl Pts',(-1.48751289001078,5.86890020544803,9.03974351324414));
#63233=CARTESIAN_POINT('Ctrl Pts',(-1.28767164976426,2.44929606941102,10.6876936039675));
#63234=CARTESIAN_POINT('Ctrl Pts',(-1.03083752138013,-2.43121825419115,
10.6868992575839));
#63235=CARTESIAN_POINT('Ctrl Pts',(-0.774094836015582,-6.82640924735232,
8.57182122854547));
#63236=CARTESIAN_POINT('Ctrl Pts',(-0.517428636590572,-9.86675985217741,
4.75781809857857));
#63237=CARTESIAN_POINT('Ctrl Pts',(-0.260829431273375,-10.9514117086836,
0.00504714446565881));
#63238=CARTESIAN_POINT('Ctrl Pts',(-0.00427994114409397,-9.86686153589834,
-4.74799752907425));
#63239=CARTESIAN_POINT('Ctrl Pts',(0.209477030133823,-7.33380134185567,
-7.92225761692041));
#63240=CARTESIAN_POINT('Ctrl Pts',(0.380470781566099,-4.63300634635791,
-9.61637377023796));
#63241=CARTESIAN_POINT('Ctrl Pts',(0.551457441280128,-1.62450730338498,
-10.6716406274424));
#63242=CARTESIAN_POINT('Ctrl Pts',(0.765180641413356,2.43544556613168,-10.6728558702936));
#63243=CARTESIAN_POINT('Ctrl Pts',(1.02165026761106,6.82783061592847,-8.55778083035606));
#63244=CARTESIAN_POINT('Ctrl Pts',(1.27813102224132,9.86352480724084,-4.74819843566146));
#63245=CARTESIAN_POINT('Ctrl Pts',(1.56313651150202,11.0772375739532,0.532638737281799));
#63246=CARTESIAN_POINT('Ctrl Pts',(1.8766998993098,9.28760209391739,6.33834310175836));
#63247=CARTESIAN_POINT('Ctrl Pts',(2.21886909367739,4.10188743890763,10.4702862968775));
#63248=CARTESIAN_POINT('Ctrl Pts',(2.56116042531579,-2.51158893027609,10.966193922874));
#63249=CARTESIAN_POINT('Ctrl Pts',(2.90361377532428,-8.25466119657915,7.65060657153079));
#63250=CARTESIAN_POINT('Ctrl Pts',(3.24625901396941,-11.1425949229273,1.66715126822539));
#63251=CARTESIAN_POINT('Ctrl Pts',(3.53197933085045,-10.3132181039043,-3.80246223862247));
#63252=CARTESIAN_POINT('Ctrl Pts',(3.81785656818665,-7.29245349613011,-8.23289553288844));
#63253=CARTESIAN_POINT('Ctrl Pts',(4.07529235944329,-2.98044886201398,-10.726822682243));
#63254=CARTESIAN_POINT('Ctrl Pts',(4.36154951821464,2.46446136838667,-10.7184995863623));
#63255=CARTESIAN_POINT('Ctrl Pts',(4.61935550740964,6.87674774915925,-8.59720962983951));
#63256=CARTESIAN_POINT('Ctrl Pts',(4.87734897679494,9.93138387504632,-4.76372459953767));
#63257=CARTESIAN_POINT('Ctrl Pts',(5.17858169940585,11.2154055251366,0.81693402950548));
#63258=CARTESIAN_POINT('Ctrl Pts',(5.52319110276872,8.99418327156995,7.19444176827225));
#63259=CARTESIAN_POINT('Ctrl Pts',(5.91140672757681,2.54413577000337,11.247876132119));
#63260=CARTESIAN_POINT('Ctrl Pts',(6.30017748440511,-5.03048374964069,10.3954931992179));
#63261=CARTESIAN_POINT('Ctrl Pts',(6.68954510735853,-10.432763020561,4.99777633096148));
#63262=CARTESIAN_POINT('Ctrl Pts',(7.07954892180132,-11.2903897670847,-2.60315821386011));
#63263=CARTESIAN_POINT('Ctrl Pts',(7.47022118865678,-7.21747965815942,-9.09075239737114));
#63264=CARTESIAN_POINT('Ctrl Pts',(7.86160367679631,0.0293157389431672,
-11.6302094613265));
#63265=CARTESIAN_POINT('Ctrl Pts',(8.18836008818057,6.07305731078864,-9.51067643046102));
#63266=CARTESIAN_POINT('Ctrl Pts',(8.45017202789412,9.34226240457075,-5.83317563617857));
#63267=CARTESIAN_POINT('Ctrl Pts',(8.71224807096988,11.2393094987126,-1.2869623709495));
#63268=CARTESIAN_POINT('Ctrl Pts',(9.0403378978682,10.5350241421098,5.10193081371875));
#63269=CARTESIAN_POINT('Ctrl Pts',(9.43487539495064,5.05431032876375,10.5813936281332));
#63270=CARTESIAN_POINT('Ctrl Pts',(9.78634691457013,-1.7876785094993,11.3463953829615));
#63271=CARTESIAN_POINT('Ctrl Pts',(10.0944857195819,-7.06345577776651,8.79648617998475));
#63272=CARTESIAN_POINT('Ctrl Pts',(10.358998280792,-10.19877817368,4.87114494261225));
#63273=CARTESIAN_POINT('Ctrl Pts',(10.6239497905261,-11.3183484730333,-0.0382477388943832));
#63274=CARTESIAN_POINT('Ctrl Pts',(10.8893064308135,-10.1976583163031,-4.95368746912103));
#63275=CARTESIAN_POINT('Ctrl Pts',(11.1551028378205,-7.04964451414481,-8.90293670258816));
#63276=CARTESIAN_POINT('Ctrl Pts',(11.4213273795416,-2.49231916840097,-11.099568267378));
#63277=CARTESIAN_POINT('Ctrl Pts',(11.6880226277189,2.57482727977078,-11.0990792013691));
#63278=CARTESIAN_POINT('Ctrl Pts',(11.9551548606348,7.14869677466965,-8.89770335751692));
#63279=CARTESIAN_POINT('Ctrl Pts',(12.2227507809561,10.3192851058014,-4.923781451297));
#63280=CARTESIAN_POINT('Ctrl Pts',(12.4908155555466,11.454693239686,0.0433976178169967));
#63281=CARTESIAN_POINT('Ctrl Pts',(12.7593530592786,10.3181824292637,5.0147287420611));
#63282=CARTESIAN_POINT('Ctrl Pts',(13.0732143174343,6.60660401385552,9.68752965695795));
#63283=CARTESIAN_POINT('Ctrl Pts',(13.4326981334329,-0.0391034732694524,
12.0247678504407));
#63284=CARTESIAN_POINT('Ctrl Pts',(13.8382440069182,-7.55120859904456,9.39895212335986));
#63285=CARTESIAN_POINT('Ctrl Pts',(14.2449041216069,-11.7963627755015,2.64906040860919));
#63286=CARTESIAN_POINT('Ctrl Pts',(14.6527221776558,-10.9045091416774,-5.29961988595021));
#63287=CARTESIAN_POINT('Ctrl Pts',(15.0616548396602,-5.2376856166355,-10.9731166019128));
#63288=CARTESIAN_POINT('Ctrl Pts',(15.471829200061,2.75900263637003,-11.8777086663017));
#63289=CARTESIAN_POINT('Ctrl Pts',(15.8144664683391,8.44283296966011,-8.3026767417502));
#63290=CARTESIAN_POINT('Ctrl Pts',(16.0894080251075,10.9344522487339,-3.76400044022369));
#63291=CARTESIAN_POINT('Ctrl Pts',(16.22689108617,11.363370689184,-1.26185267405424));
#63292=CARTESIAN_POINT('Ctrl Pts',(16.2957361032235,11.368084085471,0.048002140892809));
#63293=CARTESIAN_POINT('Ctrl Pts',(-5.41932283393119,11.2066320607065,-0.042087482955348));
#63294=CARTESIAN_POINT('Ctrl Pts',(-5.35137534985207,11.2019801129976,1.25069074479452));
#63295=CARTESIAN_POINT('Ctrl Pts',(-5.21590591317433,10.7792648066367,3.71609498960973));
#63296=CARTESIAN_POINT('Ctrl Pts',(-4.94473010944745,8.32199851399102,8.19258769576774));
#63297=CARTESIAN_POINT('Ctrl Pts',(-4.60678174808354,2.71605117015634,11.7185839329575));
#63298=CARTESIAN_POINT('Ctrl Pts',(-4.20200848807542,-5.17493114747134,
10.8269092912904));
#63299=CARTESIAN_POINT('Ctrl Pts',(-3.79831788923914,-10.7692241637846,
5.22634871152499));
#63300=CARTESIAN_POINT('Ctrl Pts',(-3.39554019651669,-11.6507475814523,
-2.62320453575906));
#63301=CARTESIAN_POINT('Ctrl Pts',(-2.9937247156788,-7.45642177572264,-9.29347997110535));
#63302=CARTESIAN_POINT('Ctrl Pts',(-2.59281954230867,-0.0314947741782245,
-11.8880880574117));
#63303=CARTESIAN_POINT('Ctrl Pts',(-2.20763151462572,7.09137672622204,-9.38831096546065));
#63304=CARTESIAN_POINT('Ctrl Pts',(-1.83801780398024,11.1273516583463,-3.46219474862477));
#63305=CARTESIAN_POINT('Ctrl Pts',(-1.54289134094969,11.1180669417964,2.25097185675394));
#63306=CARTESIAN_POINT('Ctrl Pts',(-1.33659549689802,9.43453563826111,5.73231011590964));
#63307=CARTESIAN_POINT('Ctrl Pts',(-1.21879423805378,8.07078426906925,7.44305473514828));
#63308=CARTESIAN_POINT('Ctrl Pts',(-1.07160989639206,6.06666256340522,9.3042532528442));
#63309=CARTESIAN_POINT('Ctrl Pts',(-0.865721126447319,2.54347562052076,
11.0016216538497));
#63310=CARTESIAN_POINT('Ctrl Pts',(-0.601366668027522,-2.47985430754189,
11.0002382352452));
#63311=CARTESIAN_POINT('Ctrl Pts',(-0.337362664902254,-6.99903814490822,
8.82485175419817));
#63312=CARTESIAN_POINT('Ctrl Pts',(-0.0736781085903364,-10.1219770993773,
4.90632513314084));
#63313=CARTESIAN_POINT('Ctrl Pts',(0.189674992112668,-11.2345321689752,
0.0284646833159565));
#63314=CARTESIAN_POINT('Ctrl Pts',(0.452713392534164,-10.1220192338548,
-4.84453573727029));
#63315=CARTESIAN_POINT('Ctrl Pts',(0.67166289107924,-7.52713561183215,-8.09544463026128));
#63316=CARTESIAN_POINT('Ctrl Pts',(0.846659961397844,-4.76311866049559,
-9.82909249637171));
#63317=CARTESIAN_POINT('Ctrl Pts',(1.02155884886147,-1.68579159229165,-10.9083821192465));
#63318=CARTESIAN_POINT('Ctrl Pts',(1.24002127021466,2.46400024803699,-10.9091007101121));
#63319=CARTESIAN_POINT('Ctrl Pts',(1.50188875307738,6.94836187168817,-8.74897629394682));
#63320=CARTESIAN_POINT('Ctrl Pts',(1.76348785755158,10.0440333746524,-4.8631934000533));
#63321=CARTESIAN_POINT('Ctrl Pts',(2.05386804068059,11.2798367272638,0.517220777416554));
#63322=CARTESIAN_POINT('Ctrl Pts',(2.3729315528289,9.4575572459586,6.4240027363545));
#63323=CARTESIAN_POINT('Ctrl Pts',(2.7205670766896,4.18824339806379,10.6206519716963));
#63324=CARTESIAN_POINT('Ctrl Pts',(3.06783538831903,-2.52100451397122,11.1220703552258));
#63325=CARTESIAN_POINT('Ctrl Pts',(3.41474007347489,-8.33749572436887,7.76230524925844));
#63326=CARTESIAN_POINT('Ctrl Pts',(3.76127533593318,-11.2565584243436,1.71039090787414));
#63327=CARTESIAN_POINT('Ctrl Pts',(4.04979793075202,-10.4177720610343,-3.8122691837163));
#63328=CARTESIAN_POINT('Ctrl Pts',(4.33813888512292,-7.3708240398822,-8.28046921219318));
#63329=CARTESIAN_POINT('Ctrl Pts',(4.59748984245561,-3.02638582682191,-10.7917381636151));
#63330=CARTESIAN_POINT('Ctrl Pts',(4.88546721176517,2.45091539459955,-10.7826813104226));
#63331=CARTESIAN_POINT('Ctrl Pts',(5.1445304772252,6.8841451987017,-8.65056781137807));
#63332=CARTESIAN_POINT('Ctrl Pts',(5.40347503369346,9.94931917680866,-4.8029005855658));
#63333=CARTESIAN_POINT('Ctrl Pts',(5.70543829551453,11.2356366599343,0.791211519736368));
#63334=CARTESIAN_POINT('Ctrl Pts',(6.05041155649914,9.01047842727854,7.17417649627677));
#63335=CARTESIAN_POINT('Ctrl Pts',(6.43831251816865,2.56488255568998,11.221964058039));
#63336=CARTESIAN_POINT('Ctrl Pts',(6.82608149851452,-4.98922558908911,10.3695983640868));
#63337=CARTESIAN_POINT('Ctrl Pts',(7.21375130836792,-10.3658135964222,4.99423232717637));
#63338=CARTESIAN_POINT('Ctrl Pts',(7.60136603652376,-11.2158267380261,-2.55973461164996));
#63339=CARTESIAN_POINT('Ctrl Pts',(7.98897057760673,-7.1733026858818,-8.99441899699579));
#63340=CARTESIAN_POINT('Ctrl Pts',(8.37658932011228,0.00392856028059459,
-11.5071255880267));
#63341=CARTESIAN_POINT('Ctrl Pts',(8.69968664503721,5.97856800044611,-9.40978986256599));
#63342=CARTESIAN_POINT('Ctrl Pts',(8.95817703611359,9.20571407746475,-5.77898138198752));
#63343=CARTESIAN_POINT('Ctrl Pts',(9.2167056998336,11.0767826600461,-1.29431029410649));
#63344=CARTESIAN_POINT('Ctrl Pts',(9.53998065507207,10.3809719106831,5.00005882195924));
#63345=CARTESIAN_POINT('Ctrl Pts',(9.92811301733877,4.98849876033169,10.3884980338129));
#63346=CARTESIAN_POINT('Ctrl Pts',(10.2733240631819,-1.73084177545552,11.1376898201042));
#63347=CARTESIAN_POINT('Ctrl Pts',(10.5755152860084,-6.90406708108543,8.63662622633531));
#63348=CARTESIAN_POINT('Ctrl Pts',(10.8346933356035,-9.97516159898725,4.79048819392321));
#63349=CARTESIAN_POINT('Ctrl Pts',(11.0939653660262,-11.0702259099571,-0.0135751203614283));
#63350=CARTESIAN_POINT('Ctrl Pts',(11.3534266941978,-9.97385187625692,-4.81905256665219));
#63351=CARTESIAN_POINT('Ctrl Pts',(11.6130348161363,-6.8990164224985,-8.67574529438917));
#63352=CARTESIAN_POINT('Ctrl Pts',(11.8728380427865,-2.45193812959834,-10.8184872441865));
#63353=CARTESIAN_POINT('Ctrl Pts',(12.1327787286265,2.48659962412208,-10.8176046460576));
#63354=CARTESIAN_POINT('Ctrl Pts',(12.3929463229376,6.94048671101919,-8.67331817585549));
#63355=CARTESIAN_POINT('Ctrl Pts',(12.6533133617581,10.0247151711056,-4.80685928816532));
#63356=CARTESIAN_POINT('Ctrl Pts',(12.9138935700488,11.1278743123892,0.0212671221230969));
#63357=CARTESIAN_POINT('Ctrl Pts',(13.1746990466231,10.0237725509645,4.8488500652197));
#63358=CARTESIAN_POINT('Ctrl Pts',(13.4792357338148,6.42231691433516,9.38216239452379));
#63359=CARTESIAN_POINT('Ctrl Pts',(13.8277236270411,-0.0196751530098743,
11.6463691748063));
#63360=CARTESIAN_POINT('Ctrl Pts',(14.2203419461442,-7.29096552102109,9.10302117489524));
#63361=CARTESIAN_POINT('Ctrl Pts',(14.6135758516643,-11.3943036180612,2.57588820150967));
#63362=CARTESIAN_POINT('Ctrl Pts',(15.007488851134,-10.5314196001733,-5.10041524523971));
#63363=CARTESIAN_POINT('Ctrl Pts',(15.4020230740337,-5.0636124069355,-10.5732295009402));
#63364=CARTESIAN_POINT('Ctrl Pts',(15.7974191042731,2.64381940191114,-11.4427898367074));
#63365=CARTESIAN_POINT('Ctrl Pts',(16.1272780854274,8.11545700277838,-8.00135572866133));
#63366=CARTESIAN_POINT('Ctrl Pts',(16.3919825984395,10.51368582042,-3.63176898342513));
#63367=CARTESIAN_POINT('Ctrl Pts',(16.5239960017223,10.9257856408219,-1.22936672503705));
#63368=CARTESIAN_POINT('Ctrl Pts',(16.5904023640647,10.9303320773702,0.0340899081360551));
#63369=CARTESIAN_POINT('Ctrl Pts',(-5.40297363237939,11.445432490473,-0.042087482955348));
#63370=CARTESIAN_POINT('Ctrl Pts',(-5.33369696111111,11.4406895414653,1.27598004405306));
#63371=CARTESIAN_POINT('Ctrl Pts',(-5.19521862607164,11.0085774465653,3.79612986924071));
#63372=CARTESIAN_POINT('Ctrl Pts',(-4.91840015088629,8.49992872694836,8.36573269447326));
#63373=CARTESIAN_POINT('Ctrl Pts',(-4.57320339639667,2.77438806679843,11.967805106163));
#63374=CARTESIAN_POINT('Ctrl Pts',(-4.15990469688328,-5.28321395100969,
11.056569093912));
#63375=CARTESIAN_POINT('Ctrl Pts',(-3.747686811287,-10.9955419925911,5.33820880446098));
#63376=CARTESIAN_POINT('Ctrl Pts',(-3.33647538038886,-11.8953437286105,
-2.67607624391012));
#63377=CARTESIAN_POINT('Ctrl Pts',(-2.92629230091383,-7.61357058494829,
-9.48509907357355));
#63378=CARTESIAN_POINT('Ctrl Pts',(-2.51711411539744,-0.0352081461009456,
-12.133141923791));
#63379=CARTESIAN_POINT('Ctrl Pts',(-2.12405346851776,7.23325257089384,-9.58201967934875));
#63380=CARTESIAN_POINT('Ctrl Pts',(-1.74697035839629,11.3507348234515,-3.53593739186965));
#63381=CARTESIAN_POINT('Ctrl Pts',(-1.44594495704173,11.3410956049915,2.29151330201399));
#63382=CARTESIAN_POINT('Ctrl Pts',(-1.23555813837642,9.62414272926665,5.84190263222694));
#63383=CARTESIAN_POINT('Ctrl Pts',(-1.11543119956109,8.23345778533256,7.58643680207061));
#63384=CARTESIAN_POINT('Ctrl Pts',(-0.965350761047819,6.18988758696103,
9.48427609552777));
#63385=CARTESIAN_POINT('Ctrl Pts',(-0.755455752947343,2.59800826091561,
11.2146857757666));
#63386=CARTESIAN_POINT('Ctrl Pts',(-0.486005297879084,-2.52226170629262,
11.2131697972667));
#63387=CARTESIAN_POINT('Ctrl Pts',(-0.216964169512981,-7.12771226807027,
8.99614845847778));
#63388=CARTESIAN_POINT('Ctrl Pts',(0.051673199605982,-10.3093017586739,
5.0037967419436));
#63389=CARTESIAN_POINT('Ctrl Pts',(0.319912004204202,-11.4424452984132,
0.0352862821531482));
#63390=CARTESIAN_POINT('Ctrl Pts',(0.587759827560524,-10.3093945561263,
-4.92692882386994));
#63391=CARTESIAN_POINT('Ctrl Pts',(0.810644510337,-7.66768866486485,-8.23632315062337));
#63392=CARTESIAN_POINT('Ctrl Pts',(0.9887628738834,-4.85431418623128,-10.0009017448057));
#63393=CARTESIAN_POINT('Ctrl Pts',(1.16675569936477,-1.72248496421437,-11.0992889627176));
#63394=CARTESIAN_POINT('Ctrl Pts',(1.38901397173341,2.49959534000996,-11.0999021750131));
#63395=CARTESIAN_POINT('Ctrl Pts',(1.65535913685916,7.06073570919373,-8.90264472811187));
#63396=CARTESIAN_POINT('Ctrl Pts',(1.92134523430893,10.2082911979719,-4.95142581114747));
#63397=CARTESIAN_POINT('Ctrl Pts',(2.21649491340346,11.464268710378,0.517623581655109));
#63398=CARTESIAN_POINT('Ctrl Pts',(2.54067136572795,9.61231028484355,6.51924754582076));
#63399=CARTESIAN_POINT('Ctrl Pts',(2.89372530199723,4.26040343756882,10.7809878391944));
#63400=CARTESIAN_POINT('Ctrl Pts',(3.24620579430313,-2.5499807271206,11.2895594263092));
#63401=CARTESIAN_POINT('Ctrl Pts',(3.59813519099429,-8.45086172951072,7.88046583695986));
#63402=CARTESIAN_POINT('Ctrl Pts',(3.94952923360969,-11.4105207073045,1.7432987177926));
#63403=CARTESIAN_POINT('Ctrl Pts',(4.24193167813174,-10.5600221745821,-3.85384587814088));
#63404=CARTESIAN_POINT('Ctrl Pts',(4.53402805814432,-7.47314001623606,-8.38031426693708));
#63405=CARTESIAN_POINT('Ctrl Pts',(4.79664370266186,-3.07363708606063,-10.9230350253262));
#63406=CARTESIAN_POINT('Ctrl Pts',(5.08810557752102,2.47013445948664,-10.9134823314909));
#63407=CARTESIAN_POINT('Ctrl Pts',(5.35017440554513,6.95492422204958,-8.75633618182547));
#63408=CARTESIAN_POINT('Ctrl Pts',(5.61200361956877,10.0542035018942,-4.86537952153394));
#63409=CARTESIAN_POINT('Ctrl Pts',(5.91720482332597,11.3540414258911,0.789064544875747));
#63410=CARTESIAN_POINT('Ctrl Pts',(6.26564105547289,9.10553979339257,7.23636750926088));
#63411=CARTESIAN_POINT('Ctrl Pts',(6.65717646488775,2.59867870246558,11.321535036503));
#63412=CARTESIAN_POINT('Ctrl Pts',(7.04828730943666,-5.02094595929096,10.4607994583915));
#63413=CARTESIAN_POINT('Ctrl Pts',(7.43900933211819,-10.4395500322981,5.04208746732736));
#63414=CARTESIAN_POINT('Ctrl Pts',(7.82938055234697,-11.2946782793107,-2.56617594127693));
#63415=CARTESIAN_POINT('Ctrl Pts',(8.21943575999143,-7.22551638204153,-9.04156914965989));
#63416=CARTESIAN_POINT('Ctrl Pts',(8.60921106212656,-0.0075686889805855,
-11.5674090717167));
#63417=CARTESIAN_POINT('Ctrl Pts',(8.93382080129404,5.99528673196386,-9.45936192902959));
#63418=CARTESIAN_POINT('Ctrl Pts',(9.19340748731854,9.23614030177817,-5.81293639312917));
#63419=CARTESIAN_POINT('Ctrl Pts',(9.45293101808351,11.1142702697208,-1.3107448337562));
#63420=CARTESIAN_POINT('Ctrl Pts',(9.77723136794952,10.4154952826205,5.00401083523754));
#63421=CARTESIAN_POINT('Ctrl Pts',(10.1662605952158,5.00921490063267,10.4044353775234));
#63422=CARTESIAN_POINT('Ctrl Pts',(10.5119839322498,-1.72077939907436,11.154116840079));
#63423=CARTESIAN_POINT('Ctrl Pts',(10.8144567422258,-6.89887898300864,8.65022675987097));
#63424=CARTESIAN_POINT('Ctrl Pts',(11.0737061869649,-9.97097573622103,4.80256799145211));
#63425=CARTESIAN_POINT('Ctrl Pts',(11.332954454476,-11.0656005972151,-0.0012636146746602));
#63426=CARTESIAN_POINT('Ctrl Pts',(11.592212676988,-9.96981484505854,-4.80333442118138));
#63427=CARTESIAN_POINT('Ctrl Pts',(11.8514921790329,-6.89841951530921,-8.65513848120015));
#63428=CARTESIAN_POINT('Ctrl Pts',(12.1108041978391,-2.45923784927583,-10.7938299796143));
#63429=CARTESIAN_POINT('Ctrl Pts',(12.3701601255276,2.46836208123245,-10.7925664321256));
#63430=CARTESIAN_POINT('Ctrl Pts',(12.6295710107042,6.9094980637413,-8.65413386138286));
#63431=CARTESIAN_POINT('Ctrl Pts',(12.8890481983849,9.98316171476258,-4.8004177652554));
#63432=CARTESIAN_POINT('Ctrl Pts',(13.1486032818335,11.0817124894507,0.00909499825818533));
#63433=CARTESIAN_POINT('Ctrl Pts',(13.4082458776239,9.98216422539828,4.81540788001813));
#63434=CARTESIAN_POINT('Ctrl Pts',(13.7112804745406,6.39794424339377,9.32638055254148));
#63435=CARTESIAN_POINT('Ctrl Pts',(14.0577858522366,-0.00835395432331517,
11.5770141955486));
#63436=CARTESIAN_POINT('Ctrl Pts',(14.4478987172592,-7.23337005489467,9.04881838019601));
#63437=CARTESIAN_POINT('Ctrl Pts',(14.8383177312182,-11.3068424364633,2.56726391915326));
#63438=CARTESIAN_POINT('Ctrl Pts',(15.2291319944184,-10.4497082271469,-5.04888270590908));
#63439=CARTESIAN_POINT('Ctrl Pts',(15.6202557238013,-5.02806227013448,-10.4744930049956));
#63440=CARTESIAN_POINT('Ctrl Pts',(16.0119892870161,2.60831854215743,-11.3347514386656));
#63441=CARTESIAN_POINT('Ctrl Pts',(16.338482088023,8.02442066121112,-7.9277656209221));
#63442=CARTESIAN_POINT('Ctrl Pts',(16.6004710641513,10.3977390912262,-3.60280630418266));
#63443=CARTESIAN_POINT('Ctrl Pts',(16.7309850253063,10.8049718643827,-1.22750855798432));
#63444=CARTESIAN_POINT('Ctrl Pts',(16.796746560446,10.8094741535653,0.0236795036592751));
#63445=CARTESIAN_POINT('',(-5.40297363237939,11.445432490473,-0.042087482955348));
#63446=CARTESIAN_POINT('Origin',(-6.2,11.5,0.));
#63447=CARTESIAN_POINT('',(16.796746560446,10.8094741535653,0.0236795036592751));
#63448=CARTESIAN_POINT('Ctrl Pts',(-5.40297363237939,11.445432490473,-0.042087482955348));
#63449=CARTESIAN_POINT('Ctrl Pts',(-5.33369696111111,11.4406895414653,1.27598004405306));
#63450=CARTESIAN_POINT('Ctrl Pts',(-5.19521862607164,11.0085774465653,3.79612986924071));
#63451=CARTESIAN_POINT('Ctrl Pts',(-4.91840015088629,8.49992872694836,8.36573269447326));
#63452=CARTESIAN_POINT('Ctrl Pts',(-4.57320339639667,2.77438806679843,11.967805106163));
#63453=CARTESIAN_POINT('Ctrl Pts',(-4.15990469688328,-5.28321395100969,
11.056569093912));
#63454=CARTESIAN_POINT('Ctrl Pts',(-3.747686811287,-10.9955419925911,5.33820880446098));
#63455=CARTESIAN_POINT('Ctrl Pts',(-3.33647538038886,-11.8953437286105,
-2.67607624391012));
#63456=CARTESIAN_POINT('Ctrl Pts',(-2.92629230091383,-7.61357058494829,
-9.48509907357355));
#63457=CARTESIAN_POINT('Ctrl Pts',(-2.51711411539744,-0.0352081461009456,
-12.133141923791));
#63458=CARTESIAN_POINT('Ctrl Pts',(-2.12405346851776,7.23325257089384,-9.58201967934875));
#63459=CARTESIAN_POINT('Ctrl Pts',(-1.74697035839629,11.3507348234515,-3.53593739186965));
#63460=CARTESIAN_POINT('Ctrl Pts',(-1.44594495704173,11.3410956049915,2.29151330201399));
#63461=CARTESIAN_POINT('Ctrl Pts',(-1.23555813837642,9.62414272926665,5.84190263222694));
#63462=CARTESIAN_POINT('Ctrl Pts',(-1.11543119956109,8.23345778533256,7.58643680207061));
#63463=CARTESIAN_POINT('Ctrl Pts',(-0.965350761047819,6.18988758696103,
9.48427609552777));
#63464=CARTESIAN_POINT('Ctrl Pts',(-0.755455752947343,2.59800826091561,
11.2146857757666));
#63465=CARTESIAN_POINT('Ctrl Pts',(-0.486005297879084,-2.52226170629262,
11.2131697972667));
#63466=CARTESIAN_POINT('Ctrl Pts',(-0.216964169512981,-7.12771226807027,
8.99614845847778));
#63467=CARTESIAN_POINT('Ctrl Pts',(0.051673199605982,-10.3093017586739,
5.0037967419436));
#63468=CARTESIAN_POINT('Ctrl Pts',(0.319912004204202,-11.4424452984132,
0.0352862821531482));
#63469=CARTESIAN_POINT('Ctrl Pts',(0.587759827560524,-10.3093945561263,
-4.92692882386994));
#63470=CARTESIAN_POINT('Ctrl Pts',(0.810644510337,-7.66768866486485,-8.23632315062337));
#63471=CARTESIAN_POINT('Ctrl Pts',(0.9887628738834,-4.85431418623128,-10.0009017448057));
#63472=CARTESIAN_POINT('Ctrl Pts',(1.16675569936477,-1.72248496421437,-11.0992889627176));
#63473=CARTESIAN_POINT('Ctrl Pts',(1.38901397173341,2.49959534000996,-11.0999021750131));
#63474=CARTESIAN_POINT('Ctrl Pts',(1.65535913685916,7.06073570919373,-8.90264472811187));
#63475=CARTESIAN_POINT('Ctrl Pts',(1.92134523430893,10.2082911979719,-4.95142581114747));
#63476=CARTESIAN_POINT('Ctrl Pts',(2.21649491340346,11.464268710378,0.517623581655109));
#63477=CARTESIAN_POINT('Ctrl Pts',(2.54067136572795,9.61231028484355,6.51924754582076));
#63478=CARTESIAN_POINT('Ctrl Pts',(2.89372530199723,4.26040343756882,10.7809878391944));
#63479=CARTESIAN_POINT('Ctrl Pts',(3.24620579430313,-2.5499807271206,11.2895594263092));
#63480=CARTESIAN_POINT('Ctrl Pts',(3.59813519099429,-8.45086172951072,7.88046583695986));
#63481=CARTESIAN_POINT('Ctrl Pts',(3.94952923360969,-11.4105207073045,1.7432987177926));
#63482=CARTESIAN_POINT('Ctrl Pts',(4.24193167813174,-10.5600221745821,-3.85384587814088));
#63483=CARTESIAN_POINT('Ctrl Pts',(4.53402805814432,-7.47314001623606,-8.38031426693708));
#63484=CARTESIAN_POINT('Ctrl Pts',(4.79664370266186,-3.07363708606063,-10.9230350253262));
#63485=CARTESIAN_POINT('Ctrl Pts',(5.08810557752102,2.47013445948664,-10.9134823314909));
#63486=CARTESIAN_POINT('Ctrl Pts',(5.35017440554513,6.95492422204958,-8.75633618182547));
#63487=CARTESIAN_POINT('Ctrl Pts',(5.61200361956877,10.0542035018942,-4.86537952153394));
#63488=CARTESIAN_POINT('Ctrl Pts',(5.91720482332597,11.3540414258911,0.789064544875747));
#63489=CARTESIAN_POINT('Ctrl Pts',(6.26564105547289,9.10553979339257,7.23636750926088));
#63490=CARTESIAN_POINT('Ctrl Pts',(6.65717646488775,2.59867870246558,11.321535036503));
#63491=CARTESIAN_POINT('Ctrl Pts',(7.04828730943666,-5.02094595929096,10.4607994583915));
#63492=CARTESIAN_POINT('Ctrl Pts',(7.43900933211819,-10.4395500322981,5.04208746732736));
#63493=CARTESIAN_POINT('Ctrl Pts',(7.82938055234697,-11.2946782793107,-2.56617594127693));
#63494=CARTESIAN_POINT('Ctrl Pts',(8.21943575999143,-7.22551638204153,-9.04156914965989));
#63495=CARTESIAN_POINT('Ctrl Pts',(8.60921106212656,-0.0075686889805855,
-11.5674090717167));
#63496=CARTESIAN_POINT('Ctrl Pts',(8.93382080129404,5.99528673196386,-9.45936192902959));
#63497=CARTESIAN_POINT('Ctrl Pts',(9.19340748731854,9.23614030177817,-5.81293639312917));
#63498=CARTESIAN_POINT('Ctrl Pts',(9.45293101808351,11.1142702697208,-1.3107448337562));
#63499=CARTESIAN_POINT('Ctrl Pts',(9.77723136794952,10.4154952826205,5.00401083523754));
#63500=CARTESIAN_POINT('Ctrl Pts',(10.1662605952158,5.00921490063267,10.4044353775234));
#63501=CARTESIAN_POINT('Ctrl Pts',(10.5119839322498,-1.72077939907436,11.154116840079));
#63502=CARTESIAN_POINT('Ctrl Pts',(10.8144567422258,-6.89887898300864,8.65022675987097));
#63503=CARTESIAN_POINT('Ctrl Pts',(11.0737061869649,-9.97097573622103,4.80256799145211));
#63504=CARTESIAN_POINT('Ctrl Pts',(11.332954454476,-11.0656005972151,-0.0012636146746602));
#63505=CARTESIAN_POINT('Ctrl Pts',(11.592212676988,-9.96981484505854,-4.80333442118138));
#63506=CARTESIAN_POINT('Ctrl Pts',(11.8514921790329,-6.89841951530921,-8.65513848120015));
#63507=CARTESIAN_POINT('Ctrl Pts',(12.1108041978391,-2.45923784927583,-10.7938299796143));
#63508=CARTESIAN_POINT('Ctrl Pts',(12.3701601255276,2.46836208123245,-10.7925664321256));
#63509=CARTESIAN_POINT('Ctrl Pts',(12.6295710107042,6.9094980637413,-8.65413386138286));
#63510=CARTESIAN_POINT('Ctrl Pts',(12.8890481983849,9.98316171476258,-4.8004177652554));
#63511=CARTESIAN_POINT('Ctrl Pts',(13.1486032818335,11.0817124894507,0.00909499825818533));
#63512=CARTESIAN_POINT('Ctrl Pts',(13.4082458776239,9.98216422539828,4.81540788001813));
#63513=CARTESIAN_POINT('Ctrl Pts',(13.7112804745406,6.39794424339377,9.32638055254148));
#63514=CARTESIAN_POINT('Ctrl Pts',(14.0577858522366,-0.00835395432331517,
11.5770141955486));
#63515=CARTESIAN_POINT('Ctrl Pts',(14.4478987172592,-7.23337005489467,9.04881838019601));
#63516=CARTESIAN_POINT('Ctrl Pts',(14.8383177312182,-11.3068424364633,2.56726391915326));
#63517=CARTESIAN_POINT('Ctrl Pts',(15.2291319944184,-10.4497082271469,-5.04888270590908));
#63518=CARTESIAN_POINT('Ctrl Pts',(15.6202557238013,-5.02806227013448,-10.4744930049956));
#63519=CARTESIAN_POINT('Ctrl Pts',(16.0119892870161,2.60831854215743,-11.3347514386656));
#63520=CARTESIAN_POINT('Ctrl Pts',(16.338482088023,8.02442066121112,-7.9277656209221));
#63521=CARTESIAN_POINT('Ctrl Pts',(16.6004710641513,10.3977390912262,-3.60280630418266));
#63522=CARTESIAN_POINT('Ctrl Pts',(16.7309850253063,10.8049718643827,-1.22750855798432));
#63523=CARTESIAN_POINT('Ctrl Pts',(16.796746560446,10.8094741535653,0.0236795036592751));
#63524=CARTESIAN_POINT('Origin',(17.2,11.5,-1.69309011255336E-14));
#63525=CARTESIAN_POINT('Origin',(17.2,11.5,-1.69309011255336E-14));
#63526=CARTESIAN_POINT('Origin',(-6.2,11.5,0.));
#65548=UNCERTAINTY_MEASURE_WITH_UNIT(LENGTH_MEASURE(0.01),#65564,
'DISTANCE_ACCURACY_VALUE',
'Maximum model space distance between geometric entities at asserted c
onnectivities');
#65550=UNCERTAINTY_MEASURE_WITH_UNIT(LENGTH_MEASURE(0.01),#65564,
'DISTANCE_ACCURACY_VALUE',
'Maximum model space distance between geometric entities at asserted c
onnectivities');
#65561=(
GEOMETRIC_REPRESENTATION_CONTEXT(3)
GLOBAL_UNCERTAINTY_ASSIGNED_CONTEXT((#65548))
GLOBAL_UNIT_ASSIGNED_CONTEXT((#65564,#65566,#65567))
REPRESENTATION_CONTEXT('','3D')
);
#65563=(
GEOMETRIC_REPRESENTATION_CONTEXT(3)
GLOBAL_UNCERTAINTY_ASSIGNED_CONTEXT((#65550))
GLOBAL_UNIT_ASSIGNED_CONTEXT((#65564,#65566,#65567))
REPRESENTATION_CONTEXT('','3D')
);
#65564=(
LENGTH_UNIT()
NAMED_UNIT(*)
SI_UNIT(.MILLI.,.METRE.)
);
#65566=(
NAMED_UNIT(*)
PLANE_ANGLE_UNIT()
SI_UNIT($,.RADIAN.)
);
#65567=(
NAMED_UNIT(*)
SI_UNIT($,.STERADIAN.)
SOLID_ANGLE_UNIT()
);
#65578=SHAPE_DEFINITION_REPRESENTATION(#65590,#65623);
#65590=PRODUCT_DEFINITION_SHAPE('',$,#65636);
#65623=SHAPE_REPRESENTATION('',(#22036),#65561);
#65625=PRODUCT_DEFINITION_CONTEXT('part definition',#65663,'design');
#65636=PRODUCT_DEFINITION('2026-10-10-05-45-30-305',
'10_Clutch_Compression_Spring_d1.6',#65648,#65625);
#65648=PRODUCT_DEFINITION_FORMATION('',$,#65675);
#65663=APPLICATION_CONTEXT(
'Core Data for Automotive Mechanical Design Process');
#65664=PRODUCT_CONTEXT('part definition',#65663,'mechanical');
#65675=PRODUCT('2026-10-10-05-45-30-305',
'10_Clutch_Compression_Spring_d1.6',$,(#65664));
#65782=COLOUR_RGB('Grey',0.48,0.52,0.57);
#65783=FILL_AREA_STYLE_COLOUR('',#65782);
#65784=FILL_AREA_STYLE('',(#65783));
#65785=SURFACE_STYLE_FILL_AREA(#65784);
#65786=SURFACE_SIDE_STYLE('',(#65785));
#65787=SURFACE_STYLE_USAGE(.BOTH.,#65786);
#65788=PRESENTATION_STYLE_ASSIGNMENT((#65787));
ENDSEC;
END-ISO-10303-21;
